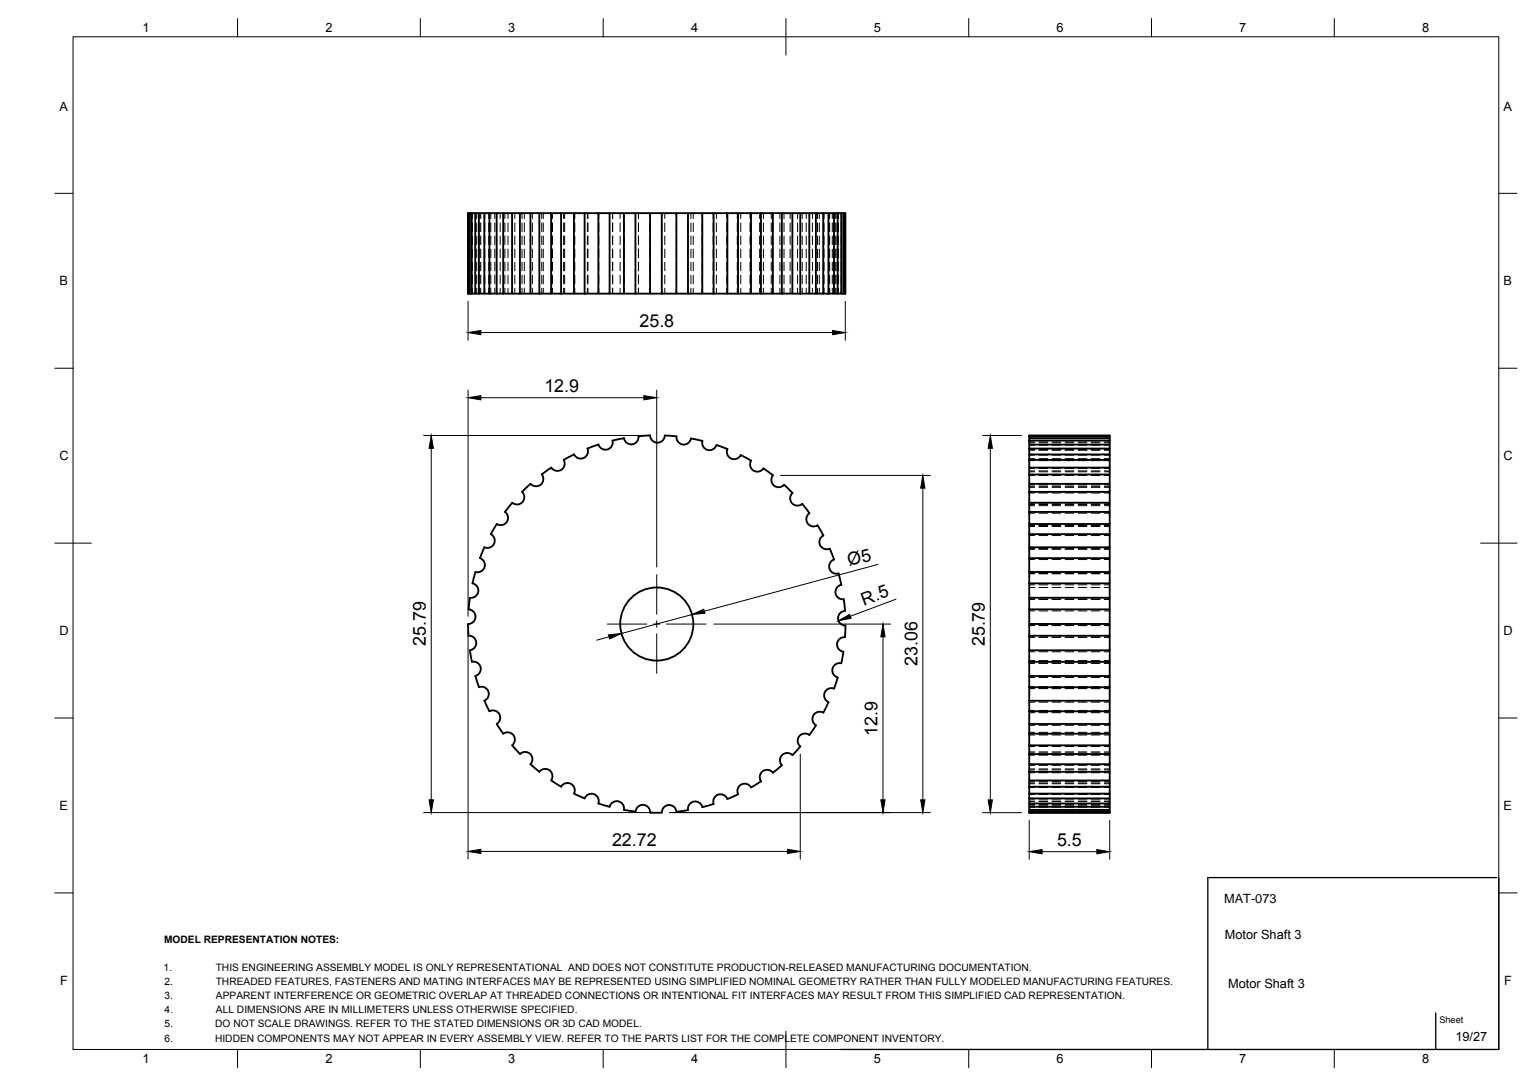
ISO-10303-21;
HEADER;
/* Generated by software containing ST-Developer
 * from STEP Tools, Inc. (www.steptools.com) 
 */

FILE_DESCRIPTION(
/* description */ ('CAx-IF Rec.Pracs.---Representation and Presentation of Product Manufa
cturing Information (PMI)---4.0---2014-10-13'),
/* implementation_level */ '2;1');

FILE_NAME(
/* name */ 'Motor Shaft 3.step',
/* time_stamp */ '2026-10-24T18:52:33-07:00',
/* author */ (''),
/* organization */ (''),
/* preprocessor_version */ 'ST-DEVELOPER v20.2',
/* originating_system */ 'Autodesk Translation Framework v15.17.0.0',
/* authorisation */ '');

FILE_SCHEMA (('AP242_MANAGED_MODEL_BASED_3D_ENGINEERING_MIM_LF { 1 0 10303 442 2 1 4 }'));
ENDSEC;

DATA;
#10=MECHANICAL_DESIGN_GEOMETRIC_PRESENTATION_REPRESENTATION('',(#434),#34876);
#368=SHAPE_REPRESENTATION_RELATIONSHIP('SRR','None',#35005,#401);
#401=ADVANCED_BREP_SHAPE_REPRESENTATION('',(#467),#34863);
#434=STYLED_ITEM('',(#35161),#467);
#467=MANIFOLD_SOLID_BREP('Motor Shaft 3',#19574);
#558=FACE_BOUND('',#6621,.T.);
#559=FACE_BOUND('',#6668,.T.);
#925=PLANE('',#21507);
#926=PLANE('',#21645);
#2083=LINE('',#32384,#3682);
#2084=LINE('',#32388,#3683);
#2085=LINE('',#32393,#3684);
#2086=LINE('',#32397,#3685);
#2087=LINE('',#32402,#3686);
#2088=LINE('',#32406,#3687);
#2089=LINE('',#32411,#3688);
#2090=LINE('',#32415,#3689);
#2091=LINE('',#32420,#3690);
#2092=LINE('',#32424,#3691);
#2093=LINE('',#32429,#3692);
#2094=LINE('',#32433,#3693);
#2095=LINE('',#32438,#3694);
#2096=LINE('',#32442,#3695);
#2097=LINE('',#32447,#3696);
#2098=LINE('',#32451,#3697);
#2099=LINE('',#32456,#3698);
#2100=LINE('',#32460,#3699);
#2101=LINE('',#32465,#3700);
#2102=LINE('',#32469,#3701);
#2103=LINE('',#32474,#3702);
#2104=LINE('',#32478,#3703);
#2105=LINE('',#32483,#3704);
#2106=LINE('',#32487,#3705);
#2107=LINE('',#32492,#3706);
#2108=LINE('',#32496,#3707);
#2109=LINE('',#32501,#3708);
#2110=LINE('',#32505,#3709);
#2111=LINE('',#32510,#3710);
#2112=LINE('',#32514,#3711);
#2113=LINE('',#32519,#3712);
#2114=LINE('',#32523,#3713);
#2115=LINE('',#32528,#3714);
#2116=LINE('',#32532,#3715);
#2117=LINE('',#32537,#3716);
#2118=LINE('',#32541,#3717);
#2119=LINE('',#32546,#3718);
#2120=LINE('',#32550,#3719);
#2121=LINE('',#32555,#3720);
#2122=LINE('',#32559,#3721);
#2123=LINE('',#32564,#3722);
#2124=LINE('',#32568,#3723);
#2125=LINE('',#32573,#3724);
#2126=LINE('',#32577,#3725);
#2127=LINE('',#32582,#3726);
#2128=LINE('',#32586,#3727);
#2129=LINE('',#32591,#3728);
#2130=LINE('',#32595,#3729);
#2131=LINE('',#32600,#3730);
#2132=LINE('',#32604,#3731);
#2133=LINE('',#32609,#3732);
#2134=LINE('',#32613,#3733);
#2135=LINE('',#32618,#3734);
#2136=LINE('',#32622,#3735);
#2137=LINE('',#32627,#3736);
#2138=LINE('',#32631,#3737);
#2139=LINE('',#32636,#3738);
#2140=LINE('',#32640,#3739);
#2141=LINE('',#32645,#3740);
#2142=LINE('',#32649,#3741);
#2143=LINE('',#32654,#3742);
#2144=LINE('',#32658,#3743);
#2145=LINE('',#32663,#3744);
#2146=LINE('',#32667,#3745);
#2147=LINE('',#32672,#3746);
#2148=LINE('',#32676,#3747);
#2149=LINE('',#32681,#3748);
#2150=LINE('',#32685,#3749);
#2151=LINE('',#32690,#3750);
#2152=LINE('',#32694,#3751);
#2153=LINE('',#32699,#3752);
#2154=LINE('',#32703,#3753);
#2155=LINE('',#32708,#3754);
#2156=LINE('',#32712,#3755);
#2157=LINE('',#32717,#3756);
#2158=LINE('',#32721,#3757);
#2159=LINE('',#32726,#3758);
#2160=LINE('',#32730,#3759);
#2161=LINE('',#32735,#3760);
#2162=LINE('',#32739,#3761);
#2163=LINE('',#32744,#3762);
#2164=LINE('',#32748,#3763);
#2165=LINE('',#32753,#3764);
#2166=LINE('',#32757,#3765);
#2167=LINE('',#32762,#3766);
#2168=LINE('',#32766,#3767);
#2169=LINE('',#32771,#3768);
#2170=LINE('',#32775,#3769);
#2171=LINE('',#32831,#3770);
#2172=LINE('',#32834,#3771);
#2173=LINE('',#32928,#3772);
#3682=VECTOR('',#26108,1.);
#3683=VECTOR('',#26111,1.);
#3684=VECTOR('',#26116,1.);
#3685=VECTOR('',#26119,1.);
#3686=VECTOR('',#26124,1.);
#3687=VECTOR('',#26127,1.);
#3688=VECTOR('',#26132,1.);
#3689=VECTOR('',#26135,1.);
#3690=VECTOR('',#26140,1.);
#3691=VECTOR('',#26143,1.);
#3692=VECTOR('',#26148,1.);
#3693=VECTOR('',#26151,1.);
#3694=VECTOR('',#26156,1.);
#3695=VECTOR('',#26159,1.);
#3696=VECTOR('',#26164,1.);
#3697=VECTOR('',#26167,1.);
#3698=VECTOR('',#26172,1.);
#3699=VECTOR('',#26175,1.);
#3700=VECTOR('',#26180,1.);
#3701=VECTOR('',#26183,1.);
#3702=VECTOR('',#26188,1.);
#3703=VECTOR('',#26191,1.);
#3704=VECTOR('',#26196,1.);
#3705=VECTOR('',#26199,1.);
#3706=VECTOR('',#26204,1.);
#3707=VECTOR('',#26207,1.);
#3708=VECTOR('',#26212,1.);
#3709=VECTOR('',#26215,1.);
#3710=VECTOR('',#26220,1.);
#3711=VECTOR('',#26223,1.);
#3712=VECTOR('',#26228,1.);
#3713=VECTOR('',#26231,1.);
#3714=VECTOR('',#26236,1.);
#3715=VECTOR('',#26239,1.);
#3716=VECTOR('',#26244,1.);
#3717=VECTOR('',#26247,1.);
#3718=VECTOR('',#26252,1.);
#3719=VECTOR('',#26255,1.);
#3720=VECTOR('',#26260,1.);
#3721=VECTOR('',#26263,1.);
#3722=VECTOR('',#26268,1.);
#3723=VECTOR('',#26271,1.);
#3724=VECTOR('',#26276,1.);
#3725=VECTOR('',#26279,1.);
#3726=VECTOR('',#26284,1.);
#3727=VECTOR('',#26287,1.);
#3728=VECTOR('',#26292,1.);
#3729=VECTOR('',#26295,1.);
#3730=VECTOR('',#26300,1.);
#3731=VECTOR('',#26303,1.);
#3732=VECTOR('',#26308,1.);
#3733=VECTOR('',#26311,1.);
#3734=VECTOR('',#26316,1.);
#3735=VECTOR('',#26319,1.);
#3736=VECTOR('',#26324,1.);
#3737=VECTOR('',#26327,1.);
#3738=VECTOR('',#26332,1.);
#3739=VECTOR('',#26335,1.);
#3740=VECTOR('',#26340,1.);
#3741=VECTOR('',#26343,1.);
#3742=VECTOR('',#26348,1.);
#3743=VECTOR('',#26351,1.);
#3744=VECTOR('',#26356,1.);
#3745=VECTOR('',#26359,1.);
#3746=VECTOR('',#26364,1.);
#3747=VECTOR('',#26367,1.);
#3748=VECTOR('',#26372,1.);
#3749=VECTOR('',#26375,1.);
#3750=VECTOR('',#26380,1.);
#3751=VECTOR('',#26383,1.);
#3752=VECTOR('',#26388,1.);
#3753=VECTOR('',#26391,1.);
#3754=VECTOR('',#26396,1.);
#3755=VECTOR('',#26399,1.);
#3756=VECTOR('',#26404,1.);
#3757=VECTOR('',#26407,1.);
#3758=VECTOR('',#26412,1.);
#3759=VECTOR('',#26415,1.);
#3760=VECTOR('',#26420,1.);
#3761=VECTOR('',#26423,1.);
#3762=VECTOR('',#26428,1.);
#3763=VECTOR('',#26431,1.);
#3764=VECTOR('',#26436,1.);
#3765=VECTOR('',#26439,1.);
#3766=VECTOR('',#26444,1.);
#3767=VECTOR('',#26447,1.);
#3768=VECTOR('',#26452,1.);
#3769=VECTOR('',#26455,1.);
#3770=VECTOR('',#26558,1.);
#3771=VECTOR('',#26561,1.);
#3772=VECTOR('',#26746,0.0025);
#4588=CYLINDRICAL_SURFACE('',#21375,0.0005);
#4589=CYLINDRICAL_SURFACE('',#21378,0.0005);
#4590=CYLINDRICAL_SURFACE('',#21381,0.0005);
#4591=CYLINDRICAL_SURFACE('',#21384,0.0005);
#4592=CYLINDRICAL_SURFACE('',#21387,0.0005);
#4593=CYLINDRICAL_SURFACE('',#21390,0.0005);
#4594=CYLINDRICAL_SURFACE('',#21393,0.0005);
#4595=CYLINDRICAL_SURFACE('',#21396,0.0005);
#4596=CYLINDRICAL_SURFACE('',#21399,0.0005);
#4597=CYLINDRICAL_SURFACE('',#21402,0.0005);
#4598=CYLINDRICAL_SURFACE('',#21405,0.0005);
#4599=CYLINDRICAL_SURFACE('',#21408,0.0005);
#4600=CYLINDRICAL_SURFACE('',#21411,0.0005);
#4601=CYLINDRICAL_SURFACE('',#21414,0.0005);
#4602=CYLINDRICAL_SURFACE('',#21417,0.0005);
#4603=CYLINDRICAL_SURFACE('',#21420,0.0005);
#4604=CYLINDRICAL_SURFACE('',#21423,0.0005);
#4605=CYLINDRICAL_SURFACE('',#21426,0.0005);
#4606=CYLINDRICAL_SURFACE('',#21429,0.0005);
#4607=CYLINDRICAL_SURFACE('',#21432,0.0005);
#4608=CYLINDRICAL_SURFACE('',#21435,0.0005);
#4609=CYLINDRICAL_SURFACE('',#21438,0.0005);
#4610=CYLINDRICAL_SURFACE('',#21441,0.0005);
#4611=CYLINDRICAL_SURFACE('',#21444,0.0005);
#4612=CYLINDRICAL_SURFACE('',#21447,0.0005);
#4613=CYLINDRICAL_SURFACE('',#21450,0.0005);
#4614=CYLINDRICAL_SURFACE('',#21453,0.0005);
#4615=CYLINDRICAL_SURFACE('',#21456,0.0005);
#4616=CYLINDRICAL_SURFACE('',#21459,0.0005);
#4617=CYLINDRICAL_SURFACE('',#21462,0.0005);
#4618=CYLINDRICAL_SURFACE('',#21465,0.0005);
#4619=CYLINDRICAL_SURFACE('',#21468,0.0005);
#4620=CYLINDRICAL_SURFACE('',#21471,0.0005);
#4621=CYLINDRICAL_SURFACE('',#21474,0.0005);
#4622=CYLINDRICAL_SURFACE('',#21477,0.0005);
#4623=CYLINDRICAL_SURFACE('',#21480,0.0005);
#4624=CYLINDRICAL_SURFACE('',#21483,0.0005);
#4625=CYLINDRICAL_SURFACE('',#21486,0.0005);
#4626=CYLINDRICAL_SURFACE('',#21489,0.0005);
#4627=CYLINDRICAL_SURFACE('',#21492,0.0005);
#4628=CYLINDRICAL_SURFACE('',#21495,0.0005);
#4629=CYLINDRICAL_SURFACE('',#21498,0.0005);
#4630=CYLINDRICAL_SURFACE('',#21501,0.0005);
#4631=CYLINDRICAL_SURFACE('',#21504,0.0005);
#4632=CYLINDRICAL_SURFACE('',#21555,0.0129);
#4633=CYLINDRICAL_SURFACE('',#21557,0.0129);
#4634=CYLINDRICAL_SURFACE('',#21559,0.0129);
#4635=CYLINDRICAL_SURFACE('',#21561,0.0129);
#4636=CYLINDRICAL_SURFACE('',#21563,0.0129);
#4637=CYLINDRICAL_SURFACE('',#21565,0.0129);
#4638=CYLINDRICAL_SURFACE('',#21567,0.0129);
#4639=CYLINDRICAL_SURFACE('',#21569,0.0129);
#4640=CYLINDRICAL_SURFACE('',#21571,0.0129);
#4641=CYLINDRICAL_SURFACE('',#21573,0.0129);
#4642=CYLINDRICAL_SURFACE('',#21575,0.0129);
#4643=CYLINDRICAL_SURFACE('',#21577,0.0129);
#4644=CYLINDRICAL_SURFACE('',#21579,0.0129);
#4645=CYLINDRICAL_SURFACE('',#21581,0.0129);
#4646=CYLINDRICAL_SURFACE('',#21583,0.0129);
#4647=CYLINDRICAL_SURFACE('',#21585,0.0129);
#4648=CYLINDRICAL_SURFACE('',#21587,0.0129);
#4649=CYLINDRICAL_SURFACE('',#21589,0.0129);
#4650=CYLINDRICAL_SURFACE('',#21591,0.0129);
#4651=CYLINDRICAL_SURFACE('',#21593,0.0129);
#4652=CYLINDRICAL_SURFACE('',#21595,0.0129);
#4653=CYLINDRICAL_SURFACE('',#21597,0.0129);
#4654=CYLINDRICAL_SURFACE('',#21599,0.0129);
#4655=CYLINDRICAL_SURFACE('',#21601,0.0129);
#4656=CYLINDRICAL_SURFACE('',#21603,0.0129);
#4657=CYLINDRICAL_SURFACE('',#21605,0.0129);
#4658=CYLINDRICAL_SURFACE('',#21607,0.0129);
#4659=CYLINDRICAL_SURFACE('',#21609,0.0129);
#4660=CYLINDRICAL_SURFACE('',#21611,0.0129);
#4661=CYLINDRICAL_SURFACE('',#21613,0.0129);
#4662=CYLINDRICAL_SURFACE('',#21615,0.0129);
#4663=CYLINDRICAL_SURFACE('',#21617,0.0129);
#4664=CYLINDRICAL_SURFACE('',#21619,0.0129);
#4665=CYLINDRICAL_SURFACE('',#21621,0.0129);
#4666=CYLINDRICAL_SURFACE('',#21623,0.0129);
#4667=CYLINDRICAL_SURFACE('',#21625,0.0129);
#4668=CYLINDRICAL_SURFACE('',#21627,0.0129);
#4669=CYLINDRICAL_SURFACE('',#21629,0.0129);
#4670=CYLINDRICAL_SURFACE('',#21631,0.0129);
#4671=CYLINDRICAL_SURFACE('',#21633,0.0129);
#4672=CYLINDRICAL_SURFACE('',#21635,0.0129);
#4673=CYLINDRICAL_SURFACE('',#21637,0.0129);
#4674=CYLINDRICAL_SURFACE('',#21639,0.0129);
#4675=CYLINDRICAL_SURFACE('',#21641,0.0129);
#4676=CYLINDRICAL_SURFACE('',#21643,0.0005);
#4677=CYLINDRICAL_SURFACE('',#21648,0.0129);
#4678=CYLINDRICAL_SURFACE('',#21649,0.0025);
#5453=FACE_OUTER_BOUND('',#6576,.T.);
#5454=FACE_OUTER_BOUND('',#6577,.T.);
#5455=FACE_OUTER_BOUND('',#6578,.T.);
#5456=FACE_OUTER_BOUND('',#6579,.T.);
#5457=FACE_OUTER_BOUND('',#6580,.T.);
#5458=FACE_OUTER_BOUND('',#6581,.T.);
#5459=FACE_OUTER_BOUND('',#6582,.T.);
#5460=FACE_OUTER_BOUND('',#6583,.T.);
#5461=FACE_OUTER_BOUND('',#6584,.T.);
#5462=FACE_OUTER_BOUND('',#6585,.T.);
#5463=FACE_OUTER_BOUND('',#6586,.T.);
#5464=FACE_OUTER_BOUND('',#6587,.T.);
#5465=FACE_OUTER_BOUND('',#6588,.T.);
#5466=FACE_OUTER_BOUND('',#6589,.T.);
#5467=FACE_OUTER_BOUND('',#6590,.T.);
#5468=FACE_OUTER_BOUND('',#6591,.T.);
#5469=FACE_OUTER_BOUND('',#6592,.T.);
#5470=FACE_OUTER_BOUND('',#6593,.T.);
#5471=FACE_OUTER_BOUND('',#6594,.T.);
#5472=FACE_OUTER_BOUND('',#6595,.T.);
#5473=FACE_OUTER_BOUND('',#6596,.T.);
#5474=FACE_OUTER_BOUND('',#6597,.T.);
#5475=FACE_OUTER_BOUND('',#6598,.T.);
#5476=FACE_OUTER_BOUND('',#6599,.T.);
#5477=FACE_OUTER_BOUND('',#6600,.T.);
#5478=FACE_OUTER_BOUND('',#6601,.T.);
#5479=FACE_OUTER_BOUND('',#6602,.T.);
#5480=FACE_OUTER_BOUND('',#6603,.T.);
#5481=FACE_OUTER_BOUND('',#6604,.T.);
#5482=FACE_OUTER_BOUND('',#6605,.T.);
#5483=FACE_OUTER_BOUND('',#6606,.T.);
#5484=FACE_OUTER_BOUND('',#6607,.T.);
#5485=FACE_OUTER_BOUND('',#6608,.T.);
#5486=FACE_OUTER_BOUND('',#6609,.T.);
#5487=FACE_OUTER_BOUND('',#6610,.T.);
#5488=FACE_OUTER_BOUND('',#6611,.T.);
#5489=FACE_OUTER_BOUND('',#6612,.T.);
#5490=FACE_OUTER_BOUND('',#6613,.T.);
#5491=FACE_OUTER_BOUND('',#6614,.T.);
#5492=FACE_OUTER_BOUND('',#6615,.T.);
#5493=FACE_OUTER_BOUND('',#6616,.T.);
#5494=FACE_OUTER_BOUND('',#6617,.T.);
#5495=FACE_OUTER_BOUND('',#6618,.T.);
#5496=FACE_OUTER_BOUND('',#6619,.T.);
#5497=FACE_OUTER_BOUND('',#6620,.T.);
#5498=FACE_OUTER_BOUND('',#6622,.T.);
#5499=FACE_OUTER_BOUND('',#6623,.T.);
#5500=FACE_OUTER_BOUND('',#6624,.T.);
#5501=FACE_OUTER_BOUND('',#6625,.T.);
#5502=FACE_OUTER_BOUND('',#6626,.T.);
#5503=FACE_OUTER_BOUND('',#6627,.T.);
#5504=FACE_OUTER_BOUND('',#6628,.T.);
#5505=FACE_OUTER_BOUND('',#6629,.T.);
#5506=FACE_OUTER_BOUND('',#6630,.T.);
#5507=FACE_OUTER_BOUND('',#6631,.T.);
#5508=FACE_OUTER_BOUND('',#6632,.T.);
#5509=FACE_OUTER_BOUND('',#6633,.T.);
#5510=FACE_OUTER_BOUND('',#6634,.T.);
#5511=FACE_OUTER_BOUND('',#6635,.T.);
#5512=FACE_OUTER_BOUND('',#6636,.T.);
#5513=FACE_OUTER_BOUND('',#6637,.T.);
#5514=FACE_OUTER_BOUND('',#6638,.T.);
#5515=FACE_OUTER_BOUND('',#6639,.T.);
#5516=FACE_OUTER_BOUND('',#6640,.T.);
#5517=FACE_OUTER_BOUND('',#6641,.T.);
#5518=FACE_OUTER_BOUND('',#6642,.T.);
#5519=FACE_OUTER_BOUND('',#6643,.T.);
#5520=FACE_OUTER_BOUND('',#6644,.T.);
#5521=FACE_OUTER_BOUND('',#6645,.T.);
#5522=FACE_OUTER_BOUND('',#6646,.T.);
#5523=FACE_OUTER_BOUND('',#6647,.T.);
#5524=FACE_OUTER_BOUND('',#6648,.T.);
#5525=FACE_OUTER_BOUND('',#6649,.T.);
#5526=FACE_OUTER_BOUND('',#6650,.T.);
#5527=FACE_OUTER_BOUND('',#6651,.T.);
#5528=FACE_OUTER_BOUND('',#6652,.T.);
#5529=FACE_OUTER_BOUND('',#6653,.T.);
#5530=FACE_OUTER_BOUND('',#6654,.T.);
#5531=FACE_OUTER_BOUND('',#6655,.T.);
#5532=FACE_OUTER_BOUND('',#6656,.T.);
#5533=FACE_OUTER_BOUND('',#6657,.T.);
#5534=FACE_OUTER_BOUND('',#6658,.T.);
#5535=FACE_OUTER_BOUND('',#6659,.T.);
#5536=FACE_OUTER_BOUND('',#6660,.T.);
#5537=FACE_OUTER_BOUND('',#6661,.T.);
#5538=FACE_OUTER_BOUND('',#6662,.T.);
#5539=FACE_OUTER_BOUND('',#6663,.T.);
#5540=FACE_OUTER_BOUND('',#6664,.T.);
#5541=FACE_OUTER_BOUND('',#6665,.T.);
#5542=FACE_OUTER_BOUND('',#6666,.T.);
#5543=FACE_OUTER_BOUND('',#6667,.T.);
#5544=FACE_OUTER_BOUND('',#6669,.T.);
#5545=FACE_OUTER_BOUND('',#6670,.T.);
#6576=EDGE_LOOP('',(#16334,#16335,#16336,#16337));
#6577=EDGE_LOOP('',(#16338,#16339,#16340,#16341));
#6578=EDGE_LOOP('',(#16342,#16343,#16344,#16345));
#6579=EDGE_LOOP('',(#16346,#16347,#16348,#16349));
#6580=EDGE_LOOP('',(#16350,#16351,#16352,#16353));
#6581=EDGE_LOOP('',(#16354,#16355,#16356,#16357));
#6582=EDGE_LOOP('',(#16358,#16359,#16360,#16361));
#6583=EDGE_LOOP('',(#16362,#16363,#16364,#16365));
#6584=EDGE_LOOP('',(#16366,#16367,#16368,#16369));
#6585=EDGE_LOOP('',(#16370,#16371,#16372,#16373));
#6586=EDGE_LOOP('',(#16374,#16375,#16376,#16377));
#6587=EDGE_LOOP('',(#16378,#16379,#16380,#16381));
#6588=EDGE_LOOP('',(#16382,#16383,#16384,#16385));
#6589=EDGE_LOOP('',(#16386,#16387,#16388,#16389));
#6590=EDGE_LOOP('',(#16390,#16391,#16392,#16393));
#6591=EDGE_LOOP('',(#16394,#16395,#16396,#16397));
#6592=EDGE_LOOP('',(#16398,#16399,#16400,#16401));
#6593=EDGE_LOOP('',(#16402,#16403,#16404,#16405));
#6594=EDGE_LOOP('',(#16406,#16407,#16408,#16409));
#6595=EDGE_LOOP('',(#16410,#16411,#16412,#16413));
#6596=EDGE_LOOP('',(#16414,#16415,#16416,#16417));
#6597=EDGE_LOOP('',(#16418,#16419,#16420,#16421));
#6598=EDGE_LOOP('',(#16422,#16423,#16424,#16425));
#6599=EDGE_LOOP('',(#16426,#16427,#16428,#16429));
#6600=EDGE_LOOP('',(#16430,#16431,#16432,#16433));
#6601=EDGE_LOOP('',(#16434,#16435,#16436,#16437));
#6602=EDGE_LOOP('',(#16438,#16439,#16440,#16441));
#6603=EDGE_LOOP('',(#16442,#16443,#16444,#16445));
#6604=EDGE_LOOP('',(#16446,#16447,#16448,#16449));
#6605=EDGE_LOOP('',(#16450,#16451,#16452,#16453));
#6606=EDGE_LOOP('',(#16454,#16455,#16456,#16457));
#6607=EDGE_LOOP('',(#16458,#16459,#16460,#16461));
#6608=EDGE_LOOP('',(#16462,#16463,#16464,#16465));
#6609=EDGE_LOOP('',(#16466,#16467,#16468,#16469));
#6610=EDGE_LOOP('',(#16470,#16471,#16472,#16473));
#6611=EDGE_LOOP('',(#16474,#16475,#16476,#16477));
#6612=EDGE_LOOP('',(#16478,#16479,#16480,#16481));
#6613=EDGE_LOOP('',(#16482,#16483,#16484,#16485));
#6614=EDGE_LOOP('',(#16486,#16487,#16488,#16489));
#6615=EDGE_LOOP('',(#16490,#16491,#16492,#16493));
#6616=EDGE_LOOP('',(#16494,#16495,#16496,#16497));
#6617=EDGE_LOOP('',(#16498,#16499,#16500,#16501));
#6618=EDGE_LOOP('',(#16502,#16503,#16504,#16505));
#6619=EDGE_LOOP('',(#16506,#16507,#16508,#16509));
#6620=EDGE_LOOP('',(#16510,#16511,#16512,#16513,#16514,#16515,#16516,#16517,
#16518,#16519,#16520,#16521,#16522,#16523,#16524,#16525,#16526,#16527,#16528,
#16529,#16530,#16531,#16532,#16533,#16534,#16535,#16536,#16537,#16538,#16539,
#16540,#16541,#16542,#16543,#16544,#16545,#16546,#16547,#16548,#16549,#16550,
#16551,#16552,#16553,#16554,#16555,#16556,#16557,#16558,#16559,#16560,#16561,
#16562,#16563,#16564,#16565,#16566,#16567,#16568,#16569,#16570,#16571,#16572,
#16573,#16574,#16575,#16576,#16577,#16578,#16579,#16580,#16581,#16582,#16583,
#16584,#16585,#16586,#16587,#16588,#16589,#16590,#16591,#16592,#16593,#16594,
#16595,#16596,#16597,#16598,#16599));
#6621=EDGE_LOOP('',(#16600));
#6622=EDGE_LOOP('',(#16601,#16602,#16603,#16604));
#6623=EDGE_LOOP('',(#16605,#16606,#16607,#16608));
#6624=EDGE_LOOP('',(#16609,#16610,#16611,#16612));
#6625=EDGE_LOOP('',(#16613,#16614,#16615,#16616));
#6626=EDGE_LOOP('',(#16617,#16618,#16619,#16620));
#6627=EDGE_LOOP('',(#16621,#16622,#16623,#16624));
#6628=EDGE_LOOP('',(#16625,#16626,#16627,#16628));
#6629=EDGE_LOOP('',(#16629,#16630,#16631,#16632));
#6630=EDGE_LOOP('',(#16633,#16634,#16635,#16636));
#6631=EDGE_LOOP('',(#16637,#16638,#16639,#16640));
#6632=EDGE_LOOP('',(#16641,#16642,#16643,#16644));
#6633=EDGE_LOOP('',(#16645,#16646,#16647,#16648));
#6634=EDGE_LOOP('',(#16649,#16650,#16651,#16652));
#6635=EDGE_LOOP('',(#16653,#16654,#16655,#16656));
#6636=EDGE_LOOP('',(#16657,#16658,#16659,#16660));
#6637=EDGE_LOOP('',(#16661,#16662,#16663,#16664));
#6638=EDGE_LOOP('',(#16665,#16666,#16667,#16668));
#6639=EDGE_LOOP('',(#16669,#16670,#16671,#16672));
#6640=EDGE_LOOP('',(#16673,#16674,#16675,#16676));
#6641=EDGE_LOOP('',(#16677,#16678,#16679,#16680));
#6642=EDGE_LOOP('',(#16681,#16682,#16683,#16684));
#6643=EDGE_LOOP('',(#16685,#16686,#16687,#16688));
#6644=EDGE_LOOP('',(#16689,#16690,#16691,#16692));
#6645=EDGE_LOOP('',(#16693,#16694,#16695,#16696));
#6646=EDGE_LOOP('',(#16697,#16698,#16699,#16700));
#6647=EDGE_LOOP('',(#16701,#16702,#16703,#16704));
#6648=EDGE_LOOP('',(#16705,#16706,#16707,#16708));
#6649=EDGE_LOOP('',(#16709,#16710,#16711,#16712));
#6650=EDGE_LOOP('',(#16713,#16714,#16715,#16716));
#6651=EDGE_LOOP('',(#16717,#16718,#16719,#16720));
#6652=EDGE_LOOP('',(#16721,#16722,#16723,#16724));
#6653=EDGE_LOOP('',(#16725,#16726,#16727,#16728));
#6654=EDGE_LOOP('',(#16729,#16730,#16731,#16732));
#6655=EDGE_LOOP('',(#16733,#16734,#16735,#16736));
#6656=EDGE_LOOP('',(#16737,#16738,#16739,#16740));
#6657=EDGE_LOOP('',(#16741,#16742,#16743,#16744));
#6658=EDGE_LOOP('',(#16745,#16746,#16747,#16748));
#6659=EDGE_LOOP('',(#16749,#16750,#16751,#16752));
#6660=EDGE_LOOP('',(#16753,#16754,#16755,#16756));
#6661=EDGE_LOOP('',(#16757,#16758,#16759,#16760));
#6662=EDGE_LOOP('',(#16761,#16762,#16763,#16764));
#6663=EDGE_LOOP('',(#16765,#16766,#16767,#16768));
#6664=EDGE_LOOP('',(#16769,#16770,#16771,#16772));
#6665=EDGE_LOOP('',(#16773,#16774,#16775,#16776));
#6666=EDGE_LOOP('',(#16777,#16778,#16779,#16780));
#6667=EDGE_LOOP('',(#16781,#16782,#16783,#16784,#16785,#16786,#16787,#16788,
#16789,#16790,#16791,#16792,#16793,#16794,#16795,#16796,#16797,#16798,#16799,
#16800,#16801,#16802,#16803,#16804,#16805,#16806,#16807,#16808,#16809,#16810,
#16811,#16812,#16813,#16814,#16815,#16816,#16817,#16818,#16819,#16820,#16821,
#16822,#16823,#16824,#16825,#16826,#16827,#16828,#16829,#16830,#16831,#16832,
#16833,#16834,#16835,#16836,#16837,#16838,#16839,#16840,#16841,#16842,#16843,
#16844,#16845,#16846,#16847,#16848,#16849,#16850,#16851,#16852,#16853,#16854,
#16855,#16856,#16857,#16858,#16859,#16860,#16861,#16862,#16863,#16864,#16865,
#16866,#16867,#16868,#16869,#16870));
#6668=EDGE_LOOP('',(#16871));
#6669=EDGE_LOOP('',(#16872,#16873,#16874,#16875));
#6670=EDGE_LOOP('',(#16876,#16877,#16878,#16879));
#7623=CIRCLE('',#21376,0.000500000000011295);
#7624=CIRCLE('',#21377,0.000500000000011295);
#7625=CIRCLE('',#21379,0.000500000000012369);
#7626=CIRCLE('',#21380,0.000500000000012369);
#7627=CIRCLE('',#21382,0.000500000000013203);
#7628=CIRCLE('',#21383,0.000500000000013203);
#7629=CIRCLE('',#21385,0.00050000000001378);
#7630=CIRCLE('',#21386,0.00050000000001378);
#7631=CIRCLE('',#21388,0.000500000000014088);
#7632=CIRCLE('',#21389,0.000500000000014088);
#7633=CIRCLE('',#21391,0.000500000000014123);
#7634=CIRCLE('',#21392,0.000500000000014123);
#7635=CIRCLE('',#21394,0.000500000000013882);
#7636=CIRCLE('',#21395,0.000500000000013882);
#7637=CIRCLE('',#21397,0.000500000000013372);
#7638=CIRCLE('',#21398,0.000500000000013372);
#7639=CIRCLE('',#21400,0.000500000000012601);
#7640=CIRCLE('',#21401,0.000500000000012601);
#7641=CIRCLE('',#21403,0.000500000000011585);
#7642=CIRCLE('',#21404,0.000500000000011585);
#7643=CIRCLE('',#21406,0.000500000000010343);
#7644=CIRCLE('',#21407,0.000500000000010343);
#7645=CIRCLE('',#21409,0.000500000000010991);
#7646=CIRCLE('',#21410,0.000500000000010991);
#7647=CIRCLE('',#21412,0.000500000000012122);
#7648=CIRCLE('',#21413,0.000500000000012122);
#7649=CIRCLE('',#21415,0.000500000000013018);
#7650=CIRCLE('',#21416,0.000500000000013018);
#7651=CIRCLE('',#21418,0.00050000000001366);
#7652=CIRCLE('',#21419,0.00050000000001366);
#7653=CIRCLE('',#21421,0.000500000000014037);
#7654=CIRCLE('',#21422,0.000500000000014037);
#7655=CIRCLE('',#21424,0.00050000000001414);
#7656=CIRCLE('',#21425,0.00050000000001414);
#7657=CIRCLE('',#21427,0.000500000000013968);
#7658=CIRCLE('',#21428,0.000500000000013968);
#7659=CIRCLE('',#21430,0.000500000000013524);
#7660=CIRCLE('',#21431,0.000500000000013524);
#7661=CIRCLE('',#21433,0.000500000000012817);
#7662=CIRCLE('',#21434,0.000500000000012817);
#7663=CIRCLE('',#21436,0.000500000000011861);
#7664=CIRCLE('',#21437,0.000500000000011861);
#7665=CIRCLE('',#21439,0.000500000000010673);
#7666=CIRCLE('',#21440,0.000500000000010673);
#7667=CIRCLE('',#21442,0.000500000000010673);
#7668=CIRCLE('',#21443,0.000500000000010673);
#7669=CIRCLE('',#21445,0.000500000000011861);
#7670=CIRCLE('',#21446,0.000500000000011861);
#7671=CIRCLE('',#21448,0.000500000000012817);
#7672=CIRCLE('',#21449,0.000500000000012817);
#7673=CIRCLE('',#21451,0.000500000000013524);
#7674=CIRCLE('',#21452,0.000500000000013524);
#7675=CIRCLE('',#21454,0.000500000000013968);
#7676=CIRCLE('',#21455,0.000500000000013968);
#7677=CIRCLE('',#21457,0.00050000000001414);
#7678=CIRCLE('',#21458,0.00050000000001414);
#7679=CIRCLE('',#21460,0.000500000000014037);
#7680=CIRCLE('',#21461,0.000500000000014037);
#7681=CIRCLE('',#21463,0.00050000000001366);
#7682=CIRCLE('',#21464,0.00050000000001366);
#7683=CIRCLE('',#21466,0.000500000000013018);
#7684=CIRCLE('',#21467,0.000500000000013018);
#7685=CIRCLE('',#21469,0.000500000000012122);
#7686=CIRCLE('',#21470,0.000500000000012122);
#7687=CIRCLE('',#21472,0.000500000000010991);
#7688=CIRCLE('',#21473,0.000500000000010991);
#7689=CIRCLE('',#21475,0.000500000000010343);
#7690=CIRCLE('',#21476,0.000500000000010343);
#7691=CIRCLE('',#21478,0.000500000000011585);
#7692=CIRCLE('',#21479,0.000500000000011585);
#7693=CIRCLE('',#21481,0.000500000000012601);
#7694=CIRCLE('',#21482,0.000500000000012601);
#7695=CIRCLE('',#21484,0.000500000000013372);
#7696=CIRCLE('',#21485,0.000500000000013372);
#7697=CIRCLE('',#21487,0.000500000000013882);
#7698=CIRCLE('',#21488,0.000500000000013882);
#7699=CIRCLE('',#21490,0.000500000000014123);
#7700=CIRCLE('',#21491,0.000500000000014123);
#7701=CIRCLE('',#21493,0.000500000000014088);
#7702=CIRCLE('',#21494,0.000500000000014088);
#7703=CIRCLE('',#21496,0.00050000000001378);
#7704=CIRCLE('',#21497,0.00050000000001378);
#7705=CIRCLE('',#21499,0.000500000000013203);
#7706=CIRCLE('',#21500,0.000500000000013203);
#7707=CIRCLE('',#21502,0.000500000000012369);
#7708=CIRCLE('',#21503,0.000500000000012369);
#7709=CIRCLE('',#21505,0.000500000000011295);
#7710=CIRCLE('',#21506,0.000500000000011295);
#7711=CIRCLE('',#21508,0.01290000000001);
#7712=CIRCLE('',#21509,0.00050000000001);
#7713=CIRCLE('',#21510,0.01290000000001);
#7714=CIRCLE('',#21511,0.01290000000001);
#7715=CIRCLE('',#21512,0.01290000000001);
#7716=CIRCLE('',#21513,0.01290000000001);
#7717=CIRCLE('',#21514,0.01290000000001);
#7718=CIRCLE('',#21515,0.01290000000001);
#7719=CIRCLE('',#21516,0.01290000000001);
#7720=CIRCLE('',#21517,0.01290000000001);
#7721=CIRCLE('',#21518,0.01290000000001);
#7722=CIRCLE('',#21519,0.01290000000001);
#7723=CIRCLE('',#21520,0.01290000000001);
#7724=CIRCLE('',#21521,0.01290000000001);
#7725=CIRCLE('',#21522,0.01290000000001);
#7726=CIRCLE('',#21523,0.01290000000001);
#7727=CIRCLE('',#21524,0.01290000000001);
#7728=CIRCLE('',#21525,0.01290000000001);
#7729=CIRCLE('',#21526,0.01290000000001);
#7730=CIRCLE('',#21527,0.01290000000001);
#7731=CIRCLE('',#21528,0.01290000000001);
#7732=CIRCLE('',#21529,0.01290000000001);
#7733=CIRCLE('',#21530,0.01290000000001);
#7734=CIRCLE('',#21531,0.01290000000001);
#7735=CIRCLE('',#21532,0.01290000000001);
#7736=CIRCLE('',#21533,0.01290000000001);
#7737=CIRCLE('',#21534,0.01290000000001);
#7738=CIRCLE('',#21535,0.01290000000001);
#7739=CIRCLE('',#21536,0.01290000000001);
#7740=CIRCLE('',#21537,0.01290000000001);
#7741=CIRCLE('',#21538,0.01290000000001);
#7742=CIRCLE('',#21539,0.01290000000001);
#7743=CIRCLE('',#21540,0.01290000000001);
#7744=CIRCLE('',#21541,0.01290000000001);
#7745=CIRCLE('',#21542,0.01290000000001);
#7746=CIRCLE('',#21543,0.01290000000001);
#7747=CIRCLE('',#21544,0.01290000000001);
#7748=CIRCLE('',#21545,0.01290000000001);
#7749=CIRCLE('',#21546,0.01290000000001);
#7750=CIRCLE('',#21547,0.01290000000001);
#7751=CIRCLE('',#21548,0.01290000000001);
#7752=CIRCLE('',#21549,0.01290000000001);
#7753=CIRCLE('',#21550,0.01290000000001);
#7754=CIRCLE('',#21551,0.01290000000001);
#7755=CIRCLE('',#21552,0.01290000000001);
#7756=CIRCLE('',#21553,0.01290000000001);
#7757=CIRCLE('',#21554,0.00250000000001);
#7758=CIRCLE('',#21556,0.01290000000001);
#7759=CIRCLE('',#21558,0.01290000000001);
#7760=CIRCLE('',#21560,0.01290000000001);
#7761=CIRCLE('',#21562,0.01290000000001);
#7762=CIRCLE('',#21564,0.01290000000001);
#7763=CIRCLE('',#21566,0.01290000000001);
#7764=CIRCLE('',#21568,0.01290000000001);
#7765=CIRCLE('',#21570,0.01290000000001);
#7766=CIRCLE('',#21572,0.01290000000001);
#7767=CIRCLE('',#21574,0.01290000000001);
#7768=CIRCLE('',#21576,0.01290000000001);
#7769=CIRCLE('',#21578,0.01290000000001);
#7770=CIRCLE('',#21580,0.01290000000001);
#7771=CIRCLE('',#21582,0.01290000000001);
#7772=CIRCLE('',#21584,0.01290000000001);
#7773=CIRCLE('',#21586,0.01290000000001);
#7774=CIRCLE('',#21588,0.01290000000001);
#7775=CIRCLE('',#21590,0.01290000000001);
#7776=CIRCLE('',#21592,0.01290000000001);
#7777=CIRCLE('',#21594,0.01290000000001);
#7778=CIRCLE('',#21596,0.01290000000001);
#7779=CIRCLE('',#21598,0.01290000000001);
#7780=CIRCLE('',#21600,0.01290000000001);
#7781=CIRCLE('',#21602,0.01290000000001);
#7782=CIRCLE('',#21604,0.01290000000001);
#7783=CIRCLE('',#21606,0.01290000000001);
#7784=CIRCLE('',#21608,0.01290000000001);
#7785=CIRCLE('',#21610,0.01290000000001);
#7786=CIRCLE('',#21612,0.01290000000001);
#7787=CIRCLE('',#21614,0.01290000000001);
#7788=CIRCLE('',#21616,0.01290000000001);
#7789=CIRCLE('',#21618,0.01290000000001);
#7790=CIRCLE('',#21620,0.01290000000001);
#7791=CIRCLE('',#21622,0.01290000000001);
#7792=CIRCLE('',#21624,0.01290000000001);
#7793=CIRCLE('',#21626,0.01290000000001);
#7794=CIRCLE('',#21628,0.01290000000001);
#7795=CIRCLE('',#21630,0.01290000000001);
#7796=CIRCLE('',#21632,0.01290000000001);
#7797=CIRCLE('',#21634,0.01290000000001);
#7798=CIRCLE('',#21636,0.01290000000001);
#7799=CIRCLE('',#21638,0.01290000000001);
#7800=CIRCLE('',#21640,0.01290000000001);
#7801=CIRCLE('',#21642,0.01290000000001);
#7802=CIRCLE('',#21644,0.00050000000001);
#7803=CIRCLE('',#21646,0.01290000000001);
#7804=CIRCLE('',#21647,0.00250000000001);
#9241=VERTEX_POINT('',#32382);
#9242=VERTEX_POINT('',#32383);
#9243=VERTEX_POINT('',#32385);
#9244=VERTEX_POINT('',#32387);
#9245=VERTEX_POINT('',#32391);
#9246=VERTEX_POINT('',#32392);
#9247=VERTEX_POINT('',#32394);
#9248=VERTEX_POINT('',#32396);
#9249=VERTEX_POINT('',#32400);
#9250=VERTEX_POINT('',#32401);
#9251=VERTEX_POINT('',#32403);
#9252=VERTEX_POINT('',#32405);
#9253=VERTEX_POINT('',#32409);
#9254=VERTEX_POINT('',#32410);
#9255=VERTEX_POINT('',#32412);
#9256=VERTEX_POINT('',#32414);
#9257=VERTEX_POINT('',#32418);
#9258=VERTEX_POINT('',#32419);
#9259=VERTEX_POINT('',#32421);
#9260=VERTEX_POINT('',#32423);
#9261=VERTEX_POINT('',#32427);
#9262=VERTEX_POINT('',#32428);
#9263=VERTEX_POINT('',#32430);
#9264=VERTEX_POINT('',#32432);
#9265=VERTEX_POINT('',#32436);
#9266=VERTEX_POINT('',#32437);
#9267=VERTEX_POINT('',#32439);
#9268=VERTEX_POINT('',#32441);
#9269=VERTEX_POINT('',#32445);
#9270=VERTEX_POINT('',#32446);
#9271=VERTEX_POINT('',#32448);
#9272=VERTEX_POINT('',#32450);
#9273=VERTEX_POINT('',#32454);
#9274=VERTEX_POINT('',#32455);
#9275=VERTEX_POINT('',#32457);
#9276=VERTEX_POINT('',#32459);
#9277=VERTEX_POINT('',#32463);
#9278=VERTEX_POINT('',#32464);
#9279=VERTEX_POINT('',#32466);
#9280=VERTEX_POINT('',#32468);
#9281=VERTEX_POINT('',#32472);
#9282=VERTEX_POINT('',#32473);
#9283=VERTEX_POINT('',#32475);
#9284=VERTEX_POINT('',#32477);
#9285=VERTEX_POINT('',#32481);
#9286=VERTEX_POINT('',#32482);
#9287=VERTEX_POINT('',#32484);
#9288=VERTEX_POINT('',#32486);
#9289=VERTEX_POINT('',#32490);
#9290=VERTEX_POINT('',#32491);
#9291=VERTEX_POINT('',#32493);
#9292=VERTEX_POINT('',#32495);
#9293=VERTEX_POINT('',#32499);
#9294=VERTEX_POINT('',#32500);
#9295=VERTEX_POINT('',#32502);
#9296=VERTEX_POINT('',#32504);
#9297=VERTEX_POINT('',#32508);
#9298=VERTEX_POINT('',#32509);
#9299=VERTEX_POINT('',#32511);
#9300=VERTEX_POINT('',#32513);
#9301=VERTEX_POINT('',#32517);
#9302=VERTEX_POINT('',#32518);
#9303=VERTEX_POINT('',#32520);
#9304=VERTEX_POINT('',#32522);
#9305=VERTEX_POINT('',#32526);
#9306=VERTEX_POINT('',#32527);
#9307=VERTEX_POINT('',#32529);
#9308=VERTEX_POINT('',#32531);
#9309=VERTEX_POINT('',#32535);
#9310=VERTEX_POINT('',#32536);
#9311=VERTEX_POINT('',#32538);
#9312=VERTEX_POINT('',#32540);
#9313=VERTEX_POINT('',#32544);
#9314=VERTEX_POINT('',#32545);
#9315=VERTEX_POINT('',#32547);
#9316=VERTEX_POINT('',#32549);
#9317=VERTEX_POINT('',#32553);
#9318=VERTEX_POINT('',#32554);
#9319=VERTEX_POINT('',#32556);
#9320=VERTEX_POINT('',#32558);
#9321=VERTEX_POINT('',#32562);
#9322=VERTEX_POINT('',#32563);
#9323=VERTEX_POINT('',#32565);
#9324=VERTEX_POINT('',#32567);
#9325=VERTEX_POINT('',#32571);
#9326=VERTEX_POINT('',#32572);
#9327=VERTEX_POINT('',#32574);
#9328=VERTEX_POINT('',#32576);
#9329=VERTEX_POINT('',#32580);
#9330=VERTEX_POINT('',#32581);
#9331=VERTEX_POINT('',#32583);
#9332=VERTEX_POINT('',#32585);
#9333=VERTEX_POINT('',#32589);
#9334=VERTEX_POINT('',#32590);
#9335=VERTEX_POINT('',#32592);
#9336=VERTEX_POINT('',#32594);
#9337=VERTEX_POINT('',#32598);
#9338=VERTEX_POINT('',#32599);
#9339=VERTEX_POINT('',#32601);
#9340=VERTEX_POINT('',#32603);
#9341=VERTEX_POINT('',#32607);
#9342=VERTEX_POINT('',#32608);
#9343=VERTEX_POINT('',#32610);
#9344=VERTEX_POINT('',#32612);
#9345=VERTEX_POINT('',#32616);
#9346=VERTEX_POINT('',#32617);
#9347=VERTEX_POINT('',#32619);
#9348=VERTEX_POINT('',#32621);
#9349=VERTEX_POINT('',#32625);
#9350=VERTEX_POINT('',#32626);
#9351=VERTEX_POINT('',#32628);
#9352=VERTEX_POINT('',#32630);
#9353=VERTEX_POINT('',#32634);
#9354=VERTEX_POINT('',#32635);
#9355=VERTEX_POINT('',#32637);
#9356=VERTEX_POINT('',#32639);
#9357=VERTEX_POINT('',#32643);
#9358=VERTEX_POINT('',#32644);
#9359=VERTEX_POINT('',#32646);
#9360=VERTEX_POINT('',#32648);
#9361=VERTEX_POINT('',#32652);
#9362=VERTEX_POINT('',#32653);
#9363=VERTEX_POINT('',#32655);
#9364=VERTEX_POINT('',#32657);
#9365=VERTEX_POINT('',#32661);
#9366=VERTEX_POINT('',#32662);
#9367=VERTEX_POINT('',#32664);
#9368=VERTEX_POINT('',#32666);
#9369=VERTEX_POINT('',#32670);
#9370=VERTEX_POINT('',#32671);
#9371=VERTEX_POINT('',#32673);
#9372=VERTEX_POINT('',#32675);
#9373=VERTEX_POINT('',#32679);
#9374=VERTEX_POINT('',#32680);
#9375=VERTEX_POINT('',#32682);
#9376=VERTEX_POINT('',#32684);
#9377=VERTEX_POINT('',#32688);
#9378=VERTEX_POINT('',#32689);
#9379=VERTEX_POINT('',#32691);
#9380=VERTEX_POINT('',#32693);
#9381=VERTEX_POINT('',#32697);
#9382=VERTEX_POINT('',#32698);
#9383=VERTEX_POINT('',#32700);
#9384=VERTEX_POINT('',#32702);
#9385=VERTEX_POINT('',#32706);
#9386=VERTEX_POINT('',#32707);
#9387=VERTEX_POINT('',#32709);
#9388=VERTEX_POINT('',#32711);
#9389=VERTEX_POINT('',#32715);
#9390=VERTEX_POINT('',#32716);
#9391=VERTEX_POINT('',#32718);
#9392=VERTEX_POINT('',#32720);
#9393=VERTEX_POINT('',#32724);
#9394=VERTEX_POINT('',#32725);
#9395=VERTEX_POINT('',#32727);
#9396=VERTEX_POINT('',#32729);
#9397=VERTEX_POINT('',#32733);
#9398=VERTEX_POINT('',#32734);
#9399=VERTEX_POINT('',#32736);
#9400=VERTEX_POINT('',#32738);
#9401=VERTEX_POINT('',#32742);
#9402=VERTEX_POINT('',#32743);
#9403=VERTEX_POINT('',#32745);
#9404=VERTEX_POINT('',#32747);
#9405=VERTEX_POINT('',#32751);
#9406=VERTEX_POINT('',#32752);
#9407=VERTEX_POINT('',#32754);
#9408=VERTEX_POINT('',#32756);
#9409=VERTEX_POINT('',#32760);
#9410=VERTEX_POINT('',#32761);
#9411=VERTEX_POINT('',#32763);
#9412=VERTEX_POINT('',#32765);
#9413=VERTEX_POINT('',#32769);
#9414=VERTEX_POINT('',#32770);
#9415=VERTEX_POINT('',#32772);
#9416=VERTEX_POINT('',#32774);
#9417=VERTEX_POINT('',#32778);
#9418=VERTEX_POINT('',#32780);
#9419=VERTEX_POINT('',#32826);
#9420=VERTEX_POINT('',#32829);
#9421=VERTEX_POINT('',#32833);
#9422=VERTEX_POINT('',#32924);
#11725=EDGE_CURVE('',#9241,#9242,#2083,.T.);
#11726=EDGE_CURVE('',#9243,#9241,#7623,.T.);
#11727=EDGE_CURVE('',#9244,#9243,#2084,.T.);
#11728=EDGE_CURVE('',#9242,#9244,#7624,.T.);
#11729=EDGE_CURVE('',#9245,#9246,#2085,.T.);
#11730=EDGE_CURVE('',#9247,#9245,#7625,.T.);
#11731=EDGE_CURVE('',#9248,#9247,#2086,.T.);
#11732=EDGE_CURVE('',#9246,#9248,#7626,.T.);
#11733=EDGE_CURVE('',#9249,#9250,#2087,.T.);
#11734=EDGE_CURVE('',#9251,#9249,#7627,.T.);
#11735=EDGE_CURVE('',#9252,#9251,#2088,.T.);
#11736=EDGE_CURVE('',#9250,#9252,#7628,.T.);
#11737=EDGE_CURVE('',#9253,#9254,#2089,.T.);
#11738=EDGE_CURVE('',#9255,#9253,#7629,.T.);
#11739=EDGE_CURVE('',#9256,#9255,#2090,.T.);
#11740=EDGE_CURVE('',#9254,#9256,#7630,.T.);
#11741=EDGE_CURVE('',#9257,#9258,#2091,.T.);
#11742=EDGE_CURVE('',#9259,#9257,#7631,.T.);
#11743=EDGE_CURVE('',#9260,#9259,#2092,.T.);
#11744=EDGE_CURVE('',#9258,#9260,#7632,.T.);
#11745=EDGE_CURVE('',#9261,#9262,#2093,.T.);
#11746=EDGE_CURVE('',#9263,#9261,#7633,.T.);
#11747=EDGE_CURVE('',#9264,#9263,#2094,.T.);
#11748=EDGE_CURVE('',#9262,#9264,#7634,.T.);
#11749=EDGE_CURVE('',#9265,#9266,#2095,.T.);
#11750=EDGE_CURVE('',#9267,#9265,#7635,.T.);
#11751=EDGE_CURVE('',#9268,#9267,#2096,.T.);
#11752=EDGE_CURVE('',#9266,#9268,#7636,.T.);
#11753=EDGE_CURVE('',#9269,#9270,#2097,.T.);
#11754=EDGE_CURVE('',#9271,#9269,#7637,.T.);
#11755=EDGE_CURVE('',#9272,#9271,#2098,.T.);
#11756=EDGE_CURVE('',#9270,#9272,#7638,.T.);
#11757=EDGE_CURVE('',#9273,#9274,#2099,.T.);
#11758=EDGE_CURVE('',#9275,#9273,#7639,.T.);
#11759=EDGE_CURVE('',#9276,#9275,#2100,.T.);
#11760=EDGE_CURVE('',#9274,#9276,#7640,.T.);
#11761=EDGE_CURVE('',#9277,#9278,#2101,.T.);
#11762=EDGE_CURVE('',#9279,#9277,#7641,.T.);
#11763=EDGE_CURVE('',#9280,#9279,#2102,.T.);
#11764=EDGE_CURVE('',#9278,#9280,#7642,.T.);
#11765=EDGE_CURVE('',#9281,#9282,#2103,.T.);
#11766=EDGE_CURVE('',#9283,#9281,#7643,.T.);
#11767=EDGE_CURVE('',#9284,#9283,#2104,.T.);
#11768=EDGE_CURVE('',#9282,#9284,#7644,.T.);
#11769=EDGE_CURVE('',#9285,#9286,#2105,.T.);
#11770=EDGE_CURVE('',#9287,#9285,#7645,.T.);
#11771=EDGE_CURVE('',#9288,#9287,#2106,.T.);
#11772=EDGE_CURVE('',#9286,#9288,#7646,.T.);
#11773=EDGE_CURVE('',#9289,#9290,#2107,.T.);
#11774=EDGE_CURVE('',#9291,#9289,#7647,.T.);
#11775=EDGE_CURVE('',#9292,#9291,#2108,.T.);
#11776=EDGE_CURVE('',#9290,#9292,#7648,.T.);
#11777=EDGE_CURVE('',#9293,#9294,#2109,.T.);
#11778=EDGE_CURVE('',#9295,#9293,#7649,.T.);
#11779=EDGE_CURVE('',#9296,#9295,#2110,.T.);
#11780=EDGE_CURVE('',#9294,#9296,#7650,.T.);
#11781=EDGE_CURVE('',#9297,#9298,#2111,.T.);
#11782=EDGE_CURVE('',#9299,#9297,#7651,.T.);
#11783=EDGE_CURVE('',#9300,#9299,#2112,.T.);
#11784=EDGE_CURVE('',#9298,#9300,#7652,.T.);
#11785=EDGE_CURVE('',#9301,#9302,#2113,.T.);
#11786=EDGE_CURVE('',#9303,#9301,#7653,.T.);
#11787=EDGE_CURVE('',#9304,#9303,#2114,.T.);
#11788=EDGE_CURVE('',#9302,#9304,#7654,.T.);
#11789=EDGE_CURVE('',#9305,#9306,#2115,.T.);
#11790=EDGE_CURVE('',#9307,#9305,#7655,.T.);
#11791=EDGE_CURVE('',#9308,#9307,#2116,.T.);
#11792=EDGE_CURVE('',#9306,#9308,#7656,.T.);
#11793=EDGE_CURVE('',#9309,#9310,#2117,.T.);
#11794=EDGE_CURVE('',#9311,#9309,#7657,.T.);
#11795=EDGE_CURVE('',#9312,#9311,#2118,.T.);
#11796=EDGE_CURVE('',#9310,#9312,#7658,.T.);
#11797=EDGE_CURVE('',#9313,#9314,#2119,.T.);
#11798=EDGE_CURVE('',#9315,#9313,#7659,.T.);
#11799=EDGE_CURVE('',#9316,#9315,#2120,.T.);
#11800=EDGE_CURVE('',#9314,#9316,#7660,.T.);
#11801=EDGE_CURVE('',#9317,#9318,#2121,.T.);
#11802=EDGE_CURVE('',#9319,#9317,#7661,.T.);
#11803=EDGE_CURVE('',#9320,#9319,#2122,.T.);
#11804=EDGE_CURVE('',#9318,#9320,#7662,.T.);
#11805=EDGE_CURVE('',#9321,#9322,#2123,.T.);
#11806=EDGE_CURVE('',#9323,#9321,#7663,.T.);
#11807=EDGE_CURVE('',#9324,#9323,#2124,.T.);
#11808=EDGE_CURVE('',#9322,#9324,#7664,.T.);
#11809=EDGE_CURVE('',#9325,#9326,#2125,.T.);
#11810=EDGE_CURVE('',#9327,#9325,#7665,.T.);
#11811=EDGE_CURVE('',#9328,#9327,#2126,.T.);
#11812=EDGE_CURVE('',#9326,#9328,#7666,.T.);
#11813=EDGE_CURVE('',#9329,#9330,#2127,.T.);
#11814=EDGE_CURVE('',#9331,#9329,#7667,.T.);
#11815=EDGE_CURVE('',#9332,#9331,#2128,.T.);
#11816=EDGE_CURVE('',#9330,#9332,#7668,.T.);
#11817=EDGE_CURVE('',#9333,#9334,#2129,.T.);
#11818=EDGE_CURVE('',#9335,#9333,#7669,.T.);
#11819=EDGE_CURVE('',#9336,#9335,#2130,.T.);
#11820=EDGE_CURVE('',#9334,#9336,#7670,.T.);
#11821=EDGE_CURVE('',#9337,#9338,#2131,.T.);
#11822=EDGE_CURVE('',#9339,#9337,#7671,.T.);
#11823=EDGE_CURVE('',#9340,#9339,#2132,.T.);
#11824=EDGE_CURVE('',#9338,#9340,#7672,.T.);
#11825=EDGE_CURVE('',#9341,#9342,#2133,.T.);
#11826=EDGE_CURVE('',#9343,#9341,#7673,.T.);
#11827=EDGE_CURVE('',#9344,#9343,#2134,.T.);
#11828=EDGE_CURVE('',#9342,#9344,#7674,.T.);
#11829=EDGE_CURVE('',#9345,#9346,#2135,.T.);
#11830=EDGE_CURVE('',#9347,#9345,#7675,.T.);
#11831=EDGE_CURVE('',#9348,#9347,#2136,.T.);
#11832=EDGE_CURVE('',#9346,#9348,#7676,.T.);
#11833=EDGE_CURVE('',#9349,#9350,#2137,.T.);
#11834=EDGE_CURVE('',#9351,#9349,#7677,.T.);
#11835=EDGE_CURVE('',#9352,#9351,#2138,.T.);
#11836=EDGE_CURVE('',#9350,#9352,#7678,.T.);
#11837=EDGE_CURVE('',#9353,#9354,#2139,.T.);
#11838=EDGE_CURVE('',#9355,#9353,#7679,.T.);
#11839=EDGE_CURVE('',#9356,#9355,#2140,.T.);
#11840=EDGE_CURVE('',#9354,#9356,#7680,.T.);
#11841=EDGE_CURVE('',#9357,#9358,#2141,.T.);
#11842=EDGE_CURVE('',#9359,#9357,#7681,.T.);
#11843=EDGE_CURVE('',#9360,#9359,#2142,.T.);
#11844=EDGE_CURVE('',#9358,#9360,#7682,.T.);
#11845=EDGE_CURVE('',#9361,#9362,#2143,.T.);
#11846=EDGE_CURVE('',#9363,#9361,#7683,.T.);
#11847=EDGE_CURVE('',#9364,#9363,#2144,.T.);
#11848=EDGE_CURVE('',#9362,#9364,#7684,.T.);
#11849=EDGE_CURVE('',#9365,#9366,#2145,.T.);
#11850=EDGE_CURVE('',#9367,#9365,#7685,.T.);
#11851=EDGE_CURVE('',#9368,#9367,#2146,.T.);
#11852=EDGE_CURVE('',#9366,#9368,#7686,.T.);
#11853=EDGE_CURVE('',#9369,#9370,#2147,.T.);
#11854=EDGE_CURVE('',#9371,#9369,#7687,.T.);
#11855=EDGE_CURVE('',#9372,#9371,#2148,.T.);
#11856=EDGE_CURVE('',#9370,#9372,#7688,.T.);
#11857=EDGE_CURVE('',#9373,#9374,#2149,.T.);
#11858=EDGE_CURVE('',#9375,#9373,#7689,.T.);
#11859=EDGE_CURVE('',#9376,#9375,#2150,.T.);
#11860=EDGE_CURVE('',#9374,#9376,#7690,.T.);
#11861=EDGE_CURVE('',#9377,#9378,#2151,.T.);
#11862=EDGE_CURVE('',#9379,#9377,#7691,.T.);
#11863=EDGE_CURVE('',#9380,#9379,#2152,.T.);
#11864=EDGE_CURVE('',#9378,#9380,#7692,.T.);
#11865=EDGE_CURVE('',#9381,#9382,#2153,.T.);
#11866=EDGE_CURVE('',#9383,#9381,#7693,.T.);
#11867=EDGE_CURVE('',#9384,#9383,#2154,.T.);
#11868=EDGE_CURVE('',#9382,#9384,#7694,.T.);
#11869=EDGE_CURVE('',#9385,#9386,#2155,.T.);
#11870=EDGE_CURVE('',#9387,#9385,#7695,.T.);
#11871=EDGE_CURVE('',#9388,#9387,#2156,.T.);
#11872=EDGE_CURVE('',#9386,#9388,#7696,.T.);
#11873=EDGE_CURVE('',#9389,#9390,#2157,.T.);
#11874=EDGE_CURVE('',#9391,#9389,#7697,.T.);
#11875=EDGE_CURVE('',#9392,#9391,#2158,.T.);
#11876=EDGE_CURVE('',#9390,#9392,#7698,.T.);
#11877=EDGE_CURVE('',#9393,#9394,#2159,.T.);
#11878=EDGE_CURVE('',#9395,#9393,#7699,.T.);
#11879=EDGE_CURVE('',#9396,#9395,#2160,.T.);
#11880=EDGE_CURVE('',#9394,#9396,#7700,.T.);
#11881=EDGE_CURVE('',#9397,#9398,#2161,.T.);
#11882=EDGE_CURVE('',#9399,#9397,#7701,.T.);
#11883=EDGE_CURVE('',#9400,#9399,#2162,.T.);
#11884=EDGE_CURVE('',#9398,#9400,#7702,.T.);
#11885=EDGE_CURVE('',#9401,#9402,#2163,.T.);
#11886=EDGE_CURVE('',#9403,#9401,#7703,.T.);
#11887=EDGE_CURVE('',#9404,#9403,#2164,.T.);
#11888=EDGE_CURVE('',#9402,#9404,#7704,.T.);
#11889=EDGE_CURVE('',#9405,#9406,#2165,.T.);
#11890=EDGE_CURVE('',#9407,#9405,#7705,.T.);
#11891=EDGE_CURVE('',#9408,#9407,#2166,.T.);
#11892=EDGE_CURVE('',#9406,#9408,#7706,.T.);
#11893=EDGE_CURVE('',#9409,#9410,#2167,.T.);
#11894=EDGE_CURVE('',#9411,#9409,#7707,.T.);
#11895=EDGE_CURVE('',#9412,#9411,#2168,.T.);
#11896=EDGE_CURVE('',#9410,#9412,#7708,.T.);
#11897=EDGE_CURVE('',#9413,#9414,#2169,.T.);
#11898=EDGE_CURVE('',#9415,#9413,#7709,.T.);
#11899=EDGE_CURVE('',#9416,#9415,#2170,.T.);
#11900=EDGE_CURVE('',#9414,#9416,#7710,.T.);
#11901=EDGE_CURVE('',#9241,#9417,#7711,.T.);
#11902=EDGE_CURVE('',#9417,#9418,#7712,.T.);
#11903=EDGE_CURVE('',#9418,#9415,#7713,.T.);
#11904=EDGE_CURVE('',#9413,#9411,#7714,.T.);
#11905=EDGE_CURVE('',#9409,#9407,#7715,.T.);
#11906=EDGE_CURVE('',#9405,#9403,#7716,.T.);
#11907=EDGE_CURVE('',#9401,#9399,#7717,.T.);
#11908=EDGE_CURVE('',#9397,#9395,#7718,.T.);
#11909=EDGE_CURVE('',#9393,#9391,#7719,.T.);
#11910=EDGE_CURVE('',#9389,#9387,#7720,.T.);
#11911=EDGE_CURVE('',#9385,#9383,#7721,.T.);
#11912=EDGE_CURVE('',#9381,#9379,#7722,.T.);
#11913=EDGE_CURVE('',#9377,#9375,#7723,.T.);
#11914=EDGE_CURVE('',#9373,#9371,#7724,.T.);
#11915=EDGE_CURVE('',#9369,#9367,#7725,.T.);
#11916=EDGE_CURVE('',#9365,#9363,#7726,.T.);
#11917=EDGE_CURVE('',#9361,#9359,#7727,.T.);
#11918=EDGE_CURVE('',#9357,#9355,#7728,.T.);
#11919=EDGE_CURVE('',#9353,#9351,#7729,.T.);
#11920=EDGE_CURVE('',#9349,#9347,#7730,.T.);
#11921=EDGE_CURVE('',#9345,#9343,#7731,.T.);
#11922=EDGE_CURVE('',#9341,#9339,#7732,.T.);
#11923=EDGE_CURVE('',#9337,#9335,#7733,.T.);
#11924=EDGE_CURVE('',#9333,#9331,#7734,.T.);
#11925=EDGE_CURVE('',#9329,#9327,#7735,.T.);
#11926=EDGE_CURVE('',#9325,#9323,#7736,.T.);
#11927=EDGE_CURVE('',#9321,#9319,#7737,.T.);
#11928=EDGE_CURVE('',#9317,#9315,#7738,.T.);
#11929=EDGE_CURVE('',#9313,#9311,#7739,.T.);
#11930=EDGE_CURVE('',#9309,#9307,#7740,.T.);
#11931=EDGE_CURVE('',#9305,#9303,#7741,.T.);
#11932=EDGE_CURVE('',#9301,#9299,#7742,.T.);
#11933=EDGE_CURVE('',#9297,#9295,#7743,.T.);
#11934=EDGE_CURVE('',#9293,#9291,#7744,.T.);
#11935=EDGE_CURVE('',#9289,#9287,#7745,.T.);
#11936=EDGE_CURVE('',#9285,#9283,#7746,.T.);
#11937=EDGE_CURVE('',#9281,#9279,#7747,.T.);
#11938=EDGE_CURVE('',#9277,#9275,#7748,.T.);
#11939=EDGE_CURVE('',#9273,#9271,#7749,.T.);
#11940=EDGE_CURVE('',#9269,#9267,#7750,.T.);
#11941=EDGE_CURVE('',#9265,#9263,#7751,.T.);
#11942=EDGE_CURVE('',#9261,#9259,#7752,.T.);
#11943=EDGE_CURVE('',#9257,#9255,#7753,.T.);
#11944=EDGE_CURVE('',#9253,#9251,#7754,.T.);
#11945=EDGE_CURVE('',#9249,#9247,#7755,.T.);
#11946=EDGE_CURVE('',#9245,#9243,#7756,.T.);
#11947=EDGE_CURVE('',#9419,#9419,#7757,.T.);
#11948=EDGE_CURVE('',#9242,#9420,#7758,.T.);
#11949=EDGE_CURVE('',#9420,#9417,#2171,.T.);
#11950=EDGE_CURVE('',#9418,#9421,#2172,.T.);
#11951=EDGE_CURVE('',#9421,#9416,#7759,.T.);
#11952=EDGE_CURVE('',#9414,#9412,#7760,.T.);
#11953=EDGE_CURVE('',#9410,#9408,#7761,.T.);
#11954=EDGE_CURVE('',#9406,#9404,#7762,.T.);
#11955=EDGE_CURVE('',#9402,#9400,#7763,.T.);
#11956=EDGE_CURVE('',#9398,#9396,#7764,.T.);
#11957=EDGE_CURVE('',#9394,#9392,#7765,.T.);
#11958=EDGE_CURVE('',#9390,#9388,#7766,.T.);
#11959=EDGE_CURVE('',#9386,#9384,#7767,.T.);
#11960=EDGE_CURVE('',#9382,#9380,#7768,.T.);
#11961=EDGE_CURVE('',#9378,#9376,#7769,.T.);
#11962=EDGE_CURVE('',#9374,#9372,#7770,.T.);
#11963=EDGE_CURVE('',#9370,#9368,#7771,.T.);
#11964=EDGE_CURVE('',#9366,#9364,#7772,.T.);
#11965=EDGE_CURVE('',#9362,#9360,#7773,.T.);
#11966=EDGE_CURVE('',#9358,#9356,#7774,.T.);
#11967=EDGE_CURVE('',#9354,#9352,#7775,.T.);
#11968=EDGE_CURVE('',#9350,#9348,#7776,.T.);
#11969=EDGE_CURVE('',#9346,#9344,#7777,.T.);
#11970=EDGE_CURVE('',#9342,#9340,#7778,.T.);
#11971=EDGE_CURVE('',#9338,#9336,#7779,.T.);
#11972=EDGE_CURVE('',#9334,#9332,#7780,.T.);
#11973=EDGE_CURVE('',#9330,#9328,#7781,.T.);
#11974=EDGE_CURVE('',#9326,#9324,#7782,.T.);
#11975=EDGE_CURVE('',#9322,#9320,#7783,.T.);
#11976=EDGE_CURVE('',#9318,#9316,#7784,.T.);
#11977=EDGE_CURVE('',#9314,#9312,#7785,.T.);
#11978=EDGE_CURVE('',#9310,#9308,#7786,.T.);
#11979=EDGE_CURVE('',#9306,#9304,#7787,.T.);
#11980=EDGE_CURVE('',#9302,#9300,#7788,.T.);
#11981=EDGE_CURVE('',#9298,#9296,#7789,.T.);
#11982=EDGE_CURVE('',#9294,#9292,#7790,.T.);
#11983=EDGE_CURVE('',#9290,#9288,#7791,.T.);
#11984=EDGE_CURVE('',#9286,#9284,#7792,.T.);
#11985=EDGE_CURVE('',#9282,#9280,#7793,.T.);
#11986=EDGE_CURVE('',#9278,#9276,#7794,.T.);
#11987=EDGE_CURVE('',#9274,#9272,#7795,.T.);
#11988=EDGE_CURVE('',#9270,#9268,#7796,.T.);
#11989=EDGE_CURVE('',#9266,#9264,#7797,.T.);
#11990=EDGE_CURVE('',#9262,#9260,#7798,.T.);
#11991=EDGE_CURVE('',#9258,#9256,#7799,.T.);
#11992=EDGE_CURVE('',#9254,#9252,#7800,.T.);
#11993=EDGE_CURVE('',#9250,#9248,#7801,.T.);
#11994=EDGE_CURVE('',#9421,#9420,#7802,.T.);
#11995=EDGE_CURVE('',#9246,#9244,#7803,.T.);
#11996=EDGE_CURVE('',#9422,#9422,#7804,.T.);
#11997=EDGE_CURVE('',#9422,#9419,#2173,.T.);
#16334=ORIENTED_EDGE('',*,*,#11725,.F.);
#16335=ORIENTED_EDGE('',*,*,#11726,.F.);
#16336=ORIENTED_EDGE('',*,*,#11727,.F.);
#16337=ORIENTED_EDGE('',*,*,#11728,.F.);
#16338=ORIENTED_EDGE('',*,*,#11729,.F.);
#16339=ORIENTED_EDGE('',*,*,#11730,.F.);
#16340=ORIENTED_EDGE('',*,*,#11731,.F.);
#16341=ORIENTED_EDGE('',*,*,#11732,.F.);
#16342=ORIENTED_EDGE('',*,*,#11733,.F.);
#16343=ORIENTED_EDGE('',*,*,#11734,.F.);
#16344=ORIENTED_EDGE('',*,*,#11735,.F.);
#16345=ORIENTED_EDGE('',*,*,#11736,.F.);
#16346=ORIENTED_EDGE('',*,*,#11737,.F.);
#16347=ORIENTED_EDGE('',*,*,#11738,.F.);
#16348=ORIENTED_EDGE('',*,*,#11739,.F.);
#16349=ORIENTED_EDGE('',*,*,#11740,.F.);
#16350=ORIENTED_EDGE('',*,*,#11741,.F.);
#16351=ORIENTED_EDGE('',*,*,#11742,.F.);
#16352=ORIENTED_EDGE('',*,*,#11743,.F.);
#16353=ORIENTED_EDGE('',*,*,#11744,.F.);
#16354=ORIENTED_EDGE('',*,*,#11745,.F.);
#16355=ORIENTED_EDGE('',*,*,#11746,.F.);
#16356=ORIENTED_EDGE('',*,*,#11747,.F.);
#16357=ORIENTED_EDGE('',*,*,#11748,.F.);
#16358=ORIENTED_EDGE('',*,*,#11749,.F.);
#16359=ORIENTED_EDGE('',*,*,#11750,.F.);
#16360=ORIENTED_EDGE('',*,*,#11751,.F.);
#16361=ORIENTED_EDGE('',*,*,#11752,.F.);
#16362=ORIENTED_EDGE('',*,*,#11753,.F.);
#16363=ORIENTED_EDGE('',*,*,#11754,.F.);
#16364=ORIENTED_EDGE('',*,*,#11755,.F.);
#16365=ORIENTED_EDGE('',*,*,#11756,.F.);
#16366=ORIENTED_EDGE('',*,*,#11757,.F.);
#16367=ORIENTED_EDGE('',*,*,#11758,.F.);
#16368=ORIENTED_EDGE('',*,*,#11759,.F.);
#16369=ORIENTED_EDGE('',*,*,#11760,.F.);
#16370=ORIENTED_EDGE('',*,*,#11761,.F.);
#16371=ORIENTED_EDGE('',*,*,#11762,.F.);
#16372=ORIENTED_EDGE('',*,*,#11763,.F.);
#16373=ORIENTED_EDGE('',*,*,#11764,.F.);
#16374=ORIENTED_EDGE('',*,*,#11765,.F.);
#16375=ORIENTED_EDGE('',*,*,#11766,.F.);
#16376=ORIENTED_EDGE('',*,*,#11767,.F.);
#16377=ORIENTED_EDGE('',*,*,#11768,.F.);
#16378=ORIENTED_EDGE('',*,*,#11769,.F.);
#16379=ORIENTED_EDGE('',*,*,#11770,.F.);
#16380=ORIENTED_EDGE('',*,*,#11771,.F.);
#16381=ORIENTED_EDGE('',*,*,#11772,.F.);
#16382=ORIENTED_EDGE('',*,*,#11773,.F.);
#16383=ORIENTED_EDGE('',*,*,#11774,.F.);
#16384=ORIENTED_EDGE('',*,*,#11775,.F.);
#16385=ORIENTED_EDGE('',*,*,#11776,.F.);
#16386=ORIENTED_EDGE('',*,*,#11777,.F.);
#16387=ORIENTED_EDGE('',*,*,#11778,.F.);
#16388=ORIENTED_EDGE('',*,*,#11779,.F.);
#16389=ORIENTED_EDGE('',*,*,#11780,.F.);
#16390=ORIENTED_EDGE('',*,*,#11781,.F.);
#16391=ORIENTED_EDGE('',*,*,#11782,.F.);
#16392=ORIENTED_EDGE('',*,*,#11783,.F.);
#16393=ORIENTED_EDGE('',*,*,#11784,.F.);
#16394=ORIENTED_EDGE('',*,*,#11785,.F.);
#16395=ORIENTED_EDGE('',*,*,#11786,.F.);
#16396=ORIENTED_EDGE('',*,*,#11787,.F.);
#16397=ORIENTED_EDGE('',*,*,#11788,.F.);
#16398=ORIENTED_EDGE('',*,*,#11789,.F.);
#16399=ORIENTED_EDGE('',*,*,#11790,.F.);
#16400=ORIENTED_EDGE('',*,*,#11791,.F.);
#16401=ORIENTED_EDGE('',*,*,#11792,.F.);
#16402=ORIENTED_EDGE('',*,*,#11793,.F.);
#16403=ORIENTED_EDGE('',*,*,#11794,.F.);
#16404=ORIENTED_EDGE('',*,*,#11795,.F.);
#16405=ORIENTED_EDGE('',*,*,#11796,.F.);
#16406=ORIENTED_EDGE('',*,*,#11797,.F.);
#16407=ORIENTED_EDGE('',*,*,#11798,.F.);
#16408=ORIENTED_EDGE('',*,*,#11799,.F.);
#16409=ORIENTED_EDGE('',*,*,#11800,.F.);
#16410=ORIENTED_EDGE('',*,*,#11801,.F.);
#16411=ORIENTED_EDGE('',*,*,#11802,.F.);
#16412=ORIENTED_EDGE('',*,*,#11803,.F.);
#16413=ORIENTED_EDGE('',*,*,#11804,.F.);
#16414=ORIENTED_EDGE('',*,*,#11805,.F.);
#16415=ORIENTED_EDGE('',*,*,#11806,.F.);
#16416=ORIENTED_EDGE('',*,*,#11807,.F.);
#16417=ORIENTED_EDGE('',*,*,#11808,.F.);
#16418=ORIENTED_EDGE('',*,*,#11809,.F.);
#16419=ORIENTED_EDGE('',*,*,#11810,.F.);
#16420=ORIENTED_EDGE('',*,*,#11811,.F.);
#16421=ORIENTED_EDGE('',*,*,#11812,.F.);
#16422=ORIENTED_EDGE('',*,*,#11813,.F.);
#16423=ORIENTED_EDGE('',*,*,#11814,.F.);
#16424=ORIENTED_EDGE('',*,*,#11815,.F.);
#16425=ORIENTED_EDGE('',*,*,#11816,.F.);
#16426=ORIENTED_EDGE('',*,*,#11817,.F.);
#16427=ORIENTED_EDGE('',*,*,#11818,.F.);
#16428=ORIENTED_EDGE('',*,*,#11819,.F.);
#16429=ORIENTED_EDGE('',*,*,#11820,.F.);
#16430=ORIENTED_EDGE('',*,*,#11821,.F.);
#16431=ORIENTED_EDGE('',*,*,#11822,.F.);
#16432=ORIENTED_EDGE('',*,*,#11823,.F.);
#16433=ORIENTED_EDGE('',*,*,#11824,.F.);
#16434=ORIENTED_EDGE('',*,*,#11825,.F.);
#16435=ORIENTED_EDGE('',*,*,#11826,.F.);
#16436=ORIENTED_EDGE('',*,*,#11827,.F.);
#16437=ORIENTED_EDGE('',*,*,#11828,.F.);
#16438=ORIENTED_EDGE('',*,*,#11829,.F.);
#16439=ORIENTED_EDGE('',*,*,#11830,.F.);
#16440=ORIENTED_EDGE('',*,*,#11831,.F.);
#16441=ORIENTED_EDGE('',*,*,#11832,.F.);
#16442=ORIENTED_EDGE('',*,*,#11833,.F.);
#16443=ORIENTED_EDGE('',*,*,#11834,.F.);
#16444=ORIENTED_EDGE('',*,*,#11835,.F.);
#16445=ORIENTED_EDGE('',*,*,#11836,.F.);
#16446=ORIENTED_EDGE('',*,*,#11837,.F.);
#16447=ORIENTED_EDGE('',*,*,#11838,.F.);
#16448=ORIENTED_EDGE('',*,*,#11839,.F.);
#16449=ORIENTED_EDGE('',*,*,#11840,.F.);
#16450=ORIENTED_EDGE('',*,*,#11841,.F.);
#16451=ORIENTED_EDGE('',*,*,#11842,.F.);
#16452=ORIENTED_EDGE('',*,*,#11843,.F.);
#16453=ORIENTED_EDGE('',*,*,#11844,.F.);
#16454=ORIENTED_EDGE('',*,*,#11845,.F.);
#16455=ORIENTED_EDGE('',*,*,#11846,.F.);
#16456=ORIENTED_EDGE('',*,*,#11847,.F.);
#16457=ORIENTED_EDGE('',*,*,#11848,.F.);
#16458=ORIENTED_EDGE('',*,*,#11849,.F.);
#16459=ORIENTED_EDGE('',*,*,#11850,.F.);
#16460=ORIENTED_EDGE('',*,*,#11851,.F.);
#16461=ORIENTED_EDGE('',*,*,#11852,.F.);
#16462=ORIENTED_EDGE('',*,*,#11853,.F.);
#16463=ORIENTED_EDGE('',*,*,#11854,.F.);
#16464=ORIENTED_EDGE('',*,*,#11855,.F.);
#16465=ORIENTED_EDGE('',*,*,#11856,.F.);
#16466=ORIENTED_EDGE('',*,*,#11857,.F.);
#16467=ORIENTED_EDGE('',*,*,#11858,.F.);
#16468=ORIENTED_EDGE('',*,*,#11859,.F.);
#16469=ORIENTED_EDGE('',*,*,#11860,.F.);
#16470=ORIENTED_EDGE('',*,*,#11861,.F.);
#16471=ORIENTED_EDGE('',*,*,#11862,.F.);
#16472=ORIENTED_EDGE('',*,*,#11863,.F.);
#16473=ORIENTED_EDGE('',*,*,#11864,.F.);
#16474=ORIENTED_EDGE('',*,*,#11865,.F.);
#16475=ORIENTED_EDGE('',*,*,#11866,.F.);
#16476=ORIENTED_EDGE('',*,*,#11867,.F.);
#16477=ORIENTED_EDGE('',*,*,#11868,.F.);
#16478=ORIENTED_EDGE('',*,*,#11869,.F.);
#16479=ORIENTED_EDGE('',*,*,#11870,.F.);
#16480=ORIENTED_EDGE('',*,*,#11871,.F.);
#16481=ORIENTED_EDGE('',*,*,#11872,.F.);
#16482=ORIENTED_EDGE('',*,*,#11873,.F.);
#16483=ORIENTED_EDGE('',*,*,#11874,.F.);
#16484=ORIENTED_EDGE('',*,*,#11875,.F.);
#16485=ORIENTED_EDGE('',*,*,#11876,.F.);
#16486=ORIENTED_EDGE('',*,*,#11877,.F.);
#16487=ORIENTED_EDGE('',*,*,#11878,.F.);
#16488=ORIENTED_EDGE('',*,*,#11879,.F.);
#16489=ORIENTED_EDGE('',*,*,#11880,.F.);
#16490=ORIENTED_EDGE('',*,*,#11881,.F.);
#16491=ORIENTED_EDGE('',*,*,#11882,.F.);
#16492=ORIENTED_EDGE('',*,*,#11883,.F.);
#16493=ORIENTED_EDGE('',*,*,#11884,.F.);
#16494=ORIENTED_EDGE('',*,*,#11885,.F.);
#16495=ORIENTED_EDGE('',*,*,#11886,.F.);
#16496=ORIENTED_EDGE('',*,*,#11887,.F.);
#16497=ORIENTED_EDGE('',*,*,#11888,.F.);
#16498=ORIENTED_EDGE('',*,*,#11889,.F.);
#16499=ORIENTED_EDGE('',*,*,#11890,.F.);
#16500=ORIENTED_EDGE('',*,*,#11891,.F.);
#16501=ORIENTED_EDGE('',*,*,#11892,.F.);
#16502=ORIENTED_EDGE('',*,*,#11893,.F.);
#16503=ORIENTED_EDGE('',*,*,#11894,.F.);
#16504=ORIENTED_EDGE('',*,*,#11895,.F.);
#16505=ORIENTED_EDGE('',*,*,#11896,.F.);
#16506=ORIENTED_EDGE('',*,*,#11897,.F.);
#16507=ORIENTED_EDGE('',*,*,#11898,.F.);
#16508=ORIENTED_EDGE('',*,*,#11899,.F.);
#16509=ORIENTED_EDGE('',*,*,#11900,.F.);
#16510=ORIENTED_EDGE('',*,*,#11726,.T.);
#16511=ORIENTED_EDGE('',*,*,#11901,.T.);
#16512=ORIENTED_EDGE('',*,*,#11902,.T.);
#16513=ORIENTED_EDGE('',*,*,#11903,.T.);
#16514=ORIENTED_EDGE('',*,*,#11898,.T.);
#16515=ORIENTED_EDGE('',*,*,#11904,.T.);
#16516=ORIENTED_EDGE('',*,*,#11894,.T.);
#16517=ORIENTED_EDGE('',*,*,#11905,.T.);
#16518=ORIENTED_EDGE('',*,*,#11890,.T.);
#16519=ORIENTED_EDGE('',*,*,#11906,.T.);
#16520=ORIENTED_EDGE('',*,*,#11886,.T.);
#16521=ORIENTED_EDGE('',*,*,#11907,.T.);
#16522=ORIENTED_EDGE('',*,*,#11882,.T.);
#16523=ORIENTED_EDGE('',*,*,#11908,.T.);
#16524=ORIENTED_EDGE('',*,*,#11878,.T.);
#16525=ORIENTED_EDGE('',*,*,#11909,.T.);
#16526=ORIENTED_EDGE('',*,*,#11874,.T.);
#16527=ORIENTED_EDGE('',*,*,#11910,.T.);
#16528=ORIENTED_EDGE('',*,*,#11870,.T.);
#16529=ORIENTED_EDGE('',*,*,#11911,.T.);
#16530=ORIENTED_EDGE('',*,*,#11866,.T.);
#16531=ORIENTED_EDGE('',*,*,#11912,.T.);
#16532=ORIENTED_EDGE('',*,*,#11862,.T.);
#16533=ORIENTED_EDGE('',*,*,#11913,.T.);
#16534=ORIENTED_EDGE('',*,*,#11858,.T.);
#16535=ORIENTED_EDGE('',*,*,#11914,.T.);
#16536=ORIENTED_EDGE('',*,*,#11854,.T.);
#16537=ORIENTED_EDGE('',*,*,#11915,.T.);
#16538=ORIENTED_EDGE('',*,*,#11850,.T.);
#16539=ORIENTED_EDGE('',*,*,#11916,.T.);
#16540=ORIENTED_EDGE('',*,*,#11846,.T.);
#16541=ORIENTED_EDGE('',*,*,#11917,.T.);
#16542=ORIENTED_EDGE('',*,*,#11842,.T.);
#16543=ORIENTED_EDGE('',*,*,#11918,.T.);
#16544=ORIENTED_EDGE('',*,*,#11838,.T.);
#16545=ORIENTED_EDGE('',*,*,#11919,.T.);
#16546=ORIENTED_EDGE('',*,*,#11834,.T.);
#16547=ORIENTED_EDGE('',*,*,#11920,.T.);
#16548=ORIENTED_EDGE('',*,*,#11830,.T.);
#16549=ORIENTED_EDGE('',*,*,#11921,.T.);
#16550=ORIENTED_EDGE('',*,*,#11826,.T.);
#16551=ORIENTED_EDGE('',*,*,#11922,.T.);
#16552=ORIENTED_EDGE('',*,*,#11822,.T.);
#16553=ORIENTED_EDGE('',*,*,#11923,.T.);
#16554=ORIENTED_EDGE('',*,*,#11818,.T.);
#16555=ORIENTED_EDGE('',*,*,#11924,.T.);
#16556=ORIENTED_EDGE('',*,*,#11814,.T.);
#16557=ORIENTED_EDGE('',*,*,#11925,.T.);
#16558=ORIENTED_EDGE('',*,*,#11810,.T.);
#16559=ORIENTED_EDGE('',*,*,#11926,.T.);
#16560=ORIENTED_EDGE('',*,*,#11806,.T.);
#16561=ORIENTED_EDGE('',*,*,#11927,.T.);
#16562=ORIENTED_EDGE('',*,*,#11802,.T.);
#16563=ORIENTED_EDGE('',*,*,#11928,.T.);
#16564=ORIENTED_EDGE('',*,*,#11798,.T.);
#16565=ORIENTED_EDGE('',*,*,#11929,.T.);
#16566=ORIENTED_EDGE('',*,*,#11794,.T.);
#16567=ORIENTED_EDGE('',*,*,#11930,.T.);
#16568=ORIENTED_EDGE('',*,*,#11790,.T.);
#16569=ORIENTED_EDGE('',*,*,#11931,.T.);
#16570=ORIENTED_EDGE('',*,*,#11786,.T.);
#16571=ORIENTED_EDGE('',*,*,#11932,.T.);
#16572=ORIENTED_EDGE('',*,*,#11782,.T.);
#16573=ORIENTED_EDGE('',*,*,#11933,.T.);
#16574=ORIENTED_EDGE('',*,*,#11778,.T.);
#16575=ORIENTED_EDGE('',*,*,#11934,.T.);
#16576=ORIENTED_EDGE('',*,*,#11774,.T.);
#16577=ORIENTED_EDGE('',*,*,#11935,.T.);
#16578=ORIENTED_EDGE('',*,*,#11770,.T.);
#16579=ORIENTED_EDGE('',*,*,#11936,.T.);
#16580=ORIENTED_EDGE('',*,*,#11766,.T.);
#16581=ORIENTED_EDGE('',*,*,#11937,.T.);
#16582=ORIENTED_EDGE('',*,*,#11762,.T.);
#16583=ORIENTED_EDGE('',*,*,#11938,.T.);
#16584=ORIENTED_EDGE('',*,*,#11758,.T.);
#16585=ORIENTED_EDGE('',*,*,#11939,.T.);
#16586=ORIENTED_EDGE('',*,*,#11754,.T.);
#16587=ORIENTED_EDGE('',*,*,#11940,.T.);
#16588=ORIENTED_EDGE('',*,*,#11750,.T.);
#16589=ORIENTED_EDGE('',*,*,#11941,.T.);
#16590=ORIENTED_EDGE('',*,*,#11746,.T.);
#16591=ORIENTED_EDGE('',*,*,#11942,.T.);
#16592=ORIENTED_EDGE('',*,*,#11742,.T.);
#16593=ORIENTED_EDGE('',*,*,#11943,.T.);
#16594=ORIENTED_EDGE('',*,*,#11738,.T.);
#16595=ORIENTED_EDGE('',*,*,#11944,.T.);
#16596=ORIENTED_EDGE('',*,*,#11734,.T.);
#16597=ORIENTED_EDGE('',*,*,#11945,.T.);
#16598=ORIENTED_EDGE('',*,*,#11730,.T.);
#16599=ORIENTED_EDGE('',*,*,#11946,.T.);
#16600=ORIENTED_EDGE('',*,*,#11947,.T.);
#16601=ORIENTED_EDGE('',*,*,#11725,.T.);
#16602=ORIENTED_EDGE('',*,*,#11948,.T.);
#16603=ORIENTED_EDGE('',*,*,#11949,.T.);
#16604=ORIENTED_EDGE('',*,*,#11901,.F.);
#16605=ORIENTED_EDGE('',*,*,#11899,.T.);
#16606=ORIENTED_EDGE('',*,*,#11903,.F.);
#16607=ORIENTED_EDGE('',*,*,#11950,.T.);
#16608=ORIENTED_EDGE('',*,*,#11951,.T.);
#16609=ORIENTED_EDGE('',*,*,#11895,.T.);
#16610=ORIENTED_EDGE('',*,*,#11904,.F.);
#16611=ORIENTED_EDGE('',*,*,#11897,.T.);
#16612=ORIENTED_EDGE('',*,*,#11952,.T.);
#16613=ORIENTED_EDGE('',*,*,#11891,.T.);
#16614=ORIENTED_EDGE('',*,*,#11905,.F.);
#16615=ORIENTED_EDGE('',*,*,#11893,.T.);
#16616=ORIENTED_EDGE('',*,*,#11953,.T.);
#16617=ORIENTED_EDGE('',*,*,#11887,.T.);
#16618=ORIENTED_EDGE('',*,*,#11906,.F.);
#16619=ORIENTED_EDGE('',*,*,#11889,.T.);
#16620=ORIENTED_EDGE('',*,*,#11954,.T.);
#16621=ORIENTED_EDGE('',*,*,#11883,.T.);
#16622=ORIENTED_EDGE('',*,*,#11907,.F.);
#16623=ORIENTED_EDGE('',*,*,#11885,.T.);
#16624=ORIENTED_EDGE('',*,*,#11955,.T.);
#16625=ORIENTED_EDGE('',*,*,#11879,.T.);
#16626=ORIENTED_EDGE('',*,*,#11908,.F.);
#16627=ORIENTED_EDGE('',*,*,#11881,.T.);
#16628=ORIENTED_EDGE('',*,*,#11956,.T.);
#16629=ORIENTED_EDGE('',*,*,#11875,.T.);
#16630=ORIENTED_EDGE('',*,*,#11909,.F.);
#16631=ORIENTED_EDGE('',*,*,#11877,.T.);
#16632=ORIENTED_EDGE('',*,*,#11957,.T.);
#16633=ORIENTED_EDGE('',*,*,#11871,.T.);
#16634=ORIENTED_EDGE('',*,*,#11910,.F.);
#16635=ORIENTED_EDGE('',*,*,#11873,.T.);
#16636=ORIENTED_EDGE('',*,*,#11958,.T.);
#16637=ORIENTED_EDGE('',*,*,#11867,.T.);
#16638=ORIENTED_EDGE('',*,*,#11911,.F.);
#16639=ORIENTED_EDGE('',*,*,#11869,.T.);
#16640=ORIENTED_EDGE('',*,*,#11959,.T.);
#16641=ORIENTED_EDGE('',*,*,#11863,.T.);
#16642=ORIENTED_EDGE('',*,*,#11912,.F.);
#16643=ORIENTED_EDGE('',*,*,#11865,.T.);
#16644=ORIENTED_EDGE('',*,*,#11960,.T.);
#16645=ORIENTED_EDGE('',*,*,#11859,.T.);
#16646=ORIENTED_EDGE('',*,*,#11913,.F.);
#16647=ORIENTED_EDGE('',*,*,#11861,.T.);
#16648=ORIENTED_EDGE('',*,*,#11961,.T.);
#16649=ORIENTED_EDGE('',*,*,#11855,.T.);
#16650=ORIENTED_EDGE('',*,*,#11914,.F.);
#16651=ORIENTED_EDGE('',*,*,#11857,.T.);
#16652=ORIENTED_EDGE('',*,*,#11962,.T.);
#16653=ORIENTED_EDGE('',*,*,#11851,.T.);
#16654=ORIENTED_EDGE('',*,*,#11915,.F.);
#16655=ORIENTED_EDGE('',*,*,#11853,.T.);
#16656=ORIENTED_EDGE('',*,*,#11963,.T.);
#16657=ORIENTED_EDGE('',*,*,#11847,.T.);
#16658=ORIENTED_EDGE('',*,*,#11916,.F.);
#16659=ORIENTED_EDGE('',*,*,#11849,.T.);
#16660=ORIENTED_EDGE('',*,*,#11964,.T.);
#16661=ORIENTED_EDGE('',*,*,#11843,.T.);
#16662=ORIENTED_EDGE('',*,*,#11917,.F.);
#16663=ORIENTED_EDGE('',*,*,#11845,.T.);
#16664=ORIENTED_EDGE('',*,*,#11965,.T.);
#16665=ORIENTED_EDGE('',*,*,#11839,.T.);
#16666=ORIENTED_EDGE('',*,*,#11918,.F.);
#16667=ORIENTED_EDGE('',*,*,#11841,.T.);
#16668=ORIENTED_EDGE('',*,*,#11966,.T.);
#16669=ORIENTED_EDGE('',*,*,#11835,.T.);
#16670=ORIENTED_EDGE('',*,*,#11919,.F.);
#16671=ORIENTED_EDGE('',*,*,#11837,.T.);
#16672=ORIENTED_EDGE('',*,*,#11967,.T.);
#16673=ORIENTED_EDGE('',*,*,#11831,.T.);
#16674=ORIENTED_EDGE('',*,*,#11920,.F.);
#16675=ORIENTED_EDGE('',*,*,#11833,.T.);
#16676=ORIENTED_EDGE('',*,*,#11968,.T.);
#16677=ORIENTED_EDGE('',*,*,#11827,.T.);
#16678=ORIENTED_EDGE('',*,*,#11921,.F.);
#16679=ORIENTED_EDGE('',*,*,#11829,.T.);
#16680=ORIENTED_EDGE('',*,*,#11969,.T.);
#16681=ORIENTED_EDGE('',*,*,#11823,.T.);
#16682=ORIENTED_EDGE('',*,*,#11922,.F.);
#16683=ORIENTED_EDGE('',*,*,#11825,.T.);
#16684=ORIENTED_EDGE('',*,*,#11970,.T.);
#16685=ORIENTED_EDGE('',*,*,#11819,.T.);
#16686=ORIENTED_EDGE('',*,*,#11923,.F.);
#16687=ORIENTED_EDGE('',*,*,#11821,.T.);
#16688=ORIENTED_EDGE('',*,*,#11971,.T.);
#16689=ORIENTED_EDGE('',*,*,#11815,.T.);
#16690=ORIENTED_EDGE('',*,*,#11924,.F.);
#16691=ORIENTED_EDGE('',*,*,#11817,.T.);
#16692=ORIENTED_EDGE('',*,*,#11972,.T.);
#16693=ORIENTED_EDGE('',*,*,#11811,.T.);
#16694=ORIENTED_EDGE('',*,*,#11925,.F.);
#16695=ORIENTED_EDGE('',*,*,#11813,.T.);
#16696=ORIENTED_EDGE('',*,*,#11973,.T.);
#16697=ORIENTED_EDGE('',*,*,#11807,.T.);
#16698=ORIENTED_EDGE('',*,*,#11926,.F.);
#16699=ORIENTED_EDGE('',*,*,#11809,.T.);
#16700=ORIENTED_EDGE('',*,*,#11974,.T.);
#16701=ORIENTED_EDGE('',*,*,#11803,.T.);
#16702=ORIENTED_EDGE('',*,*,#11927,.F.);
#16703=ORIENTED_EDGE('',*,*,#11805,.T.);
#16704=ORIENTED_EDGE('',*,*,#11975,.T.);
#16705=ORIENTED_EDGE('',*,*,#11799,.T.);
#16706=ORIENTED_EDGE('',*,*,#11928,.F.);
#16707=ORIENTED_EDGE('',*,*,#11801,.T.);
#16708=ORIENTED_EDGE('',*,*,#11976,.T.);
#16709=ORIENTED_EDGE('',*,*,#11795,.T.);
#16710=ORIENTED_EDGE('',*,*,#11929,.F.);
#16711=ORIENTED_EDGE('',*,*,#11797,.T.);
#16712=ORIENTED_EDGE('',*,*,#11977,.T.);
#16713=ORIENTED_EDGE('',*,*,#11791,.T.);
#16714=ORIENTED_EDGE('',*,*,#11930,.F.);
#16715=ORIENTED_EDGE('',*,*,#11793,.T.);
#16716=ORIENTED_EDGE('',*,*,#11978,.T.);
#16717=ORIENTED_EDGE('',*,*,#11787,.T.);
#16718=ORIENTED_EDGE('',*,*,#11931,.F.);
#16719=ORIENTED_EDGE('',*,*,#11789,.T.);
#16720=ORIENTED_EDGE('',*,*,#11979,.T.);
#16721=ORIENTED_EDGE('',*,*,#11783,.T.);
#16722=ORIENTED_EDGE('',*,*,#11932,.F.);
#16723=ORIENTED_EDGE('',*,*,#11785,.T.);
#16724=ORIENTED_EDGE('',*,*,#11980,.T.);
#16725=ORIENTED_EDGE('',*,*,#11779,.T.);
#16726=ORIENTED_EDGE('',*,*,#11933,.F.);
#16727=ORIENTED_EDGE('',*,*,#11781,.T.);
#16728=ORIENTED_EDGE('',*,*,#11981,.T.);
#16729=ORIENTED_EDGE('',*,*,#11775,.T.);
#16730=ORIENTED_EDGE('',*,*,#11934,.F.);
#16731=ORIENTED_EDGE('',*,*,#11777,.T.);
#16732=ORIENTED_EDGE('',*,*,#11982,.T.);
#16733=ORIENTED_EDGE('',*,*,#11771,.T.);
#16734=ORIENTED_EDGE('',*,*,#11935,.F.);
#16735=ORIENTED_EDGE('',*,*,#11773,.T.);
#16736=ORIENTED_EDGE('',*,*,#11983,.T.);
#16737=ORIENTED_EDGE('',*,*,#11767,.T.);
#16738=ORIENTED_EDGE('',*,*,#11936,.F.);
#16739=ORIENTED_EDGE('',*,*,#11769,.T.);
#16740=ORIENTED_EDGE('',*,*,#11984,.T.);
#16741=ORIENTED_EDGE('',*,*,#11763,.T.);
#16742=ORIENTED_EDGE('',*,*,#11937,.F.);
#16743=ORIENTED_EDGE('',*,*,#11765,.T.);
#16744=ORIENTED_EDGE('',*,*,#11985,.T.);
#16745=ORIENTED_EDGE('',*,*,#11759,.T.);
#16746=ORIENTED_EDGE('',*,*,#11938,.F.);
#16747=ORIENTED_EDGE('',*,*,#11761,.T.);
#16748=ORIENTED_EDGE('',*,*,#11986,.T.);
#16749=ORIENTED_EDGE('',*,*,#11755,.T.);
#16750=ORIENTED_EDGE('',*,*,#11939,.F.);
#16751=ORIENTED_EDGE('',*,*,#11757,.T.);
#16752=ORIENTED_EDGE('',*,*,#11987,.T.);
#16753=ORIENTED_EDGE('',*,*,#11751,.T.);
#16754=ORIENTED_EDGE('',*,*,#11940,.F.);
#16755=ORIENTED_EDGE('',*,*,#11753,.T.);
#16756=ORIENTED_EDGE('',*,*,#11988,.T.);
#16757=ORIENTED_EDGE('',*,*,#11747,.T.);
#16758=ORIENTED_EDGE('',*,*,#11941,.F.);
#16759=ORIENTED_EDGE('',*,*,#11749,.T.);
#16760=ORIENTED_EDGE('',*,*,#11989,.T.);
#16761=ORIENTED_EDGE('',*,*,#11743,.T.);
#16762=ORIENTED_EDGE('',*,*,#11942,.F.);
#16763=ORIENTED_EDGE('',*,*,#11745,.T.);
#16764=ORIENTED_EDGE('',*,*,#11990,.T.);
#16765=ORIENTED_EDGE('',*,*,#11739,.T.);
#16766=ORIENTED_EDGE('',*,*,#11943,.F.);
#16767=ORIENTED_EDGE('',*,*,#11741,.T.);
#16768=ORIENTED_EDGE('',*,*,#11991,.T.);
#16769=ORIENTED_EDGE('',*,*,#11735,.T.);
#16770=ORIENTED_EDGE('',*,*,#11944,.F.);
#16771=ORIENTED_EDGE('',*,*,#11737,.T.);
#16772=ORIENTED_EDGE('',*,*,#11992,.T.);
#16773=ORIENTED_EDGE('',*,*,#11731,.T.);
#16774=ORIENTED_EDGE('',*,*,#11945,.F.);
#16775=ORIENTED_EDGE('',*,*,#11733,.T.);
#16776=ORIENTED_EDGE('',*,*,#11993,.T.);
#16777=ORIENTED_EDGE('',*,*,#11950,.F.);
#16778=ORIENTED_EDGE('',*,*,#11902,.F.);
#16779=ORIENTED_EDGE('',*,*,#11949,.F.);
#16780=ORIENTED_EDGE('',*,*,#11994,.F.);
#16781=ORIENTED_EDGE('',*,*,#11728,.T.);
#16782=ORIENTED_EDGE('',*,*,#11995,.F.);
#16783=ORIENTED_EDGE('',*,*,#11732,.T.);
#16784=ORIENTED_EDGE('',*,*,#11993,.F.);
#16785=ORIENTED_EDGE('',*,*,#11736,.T.);
#16786=ORIENTED_EDGE('',*,*,#11992,.F.);
#16787=ORIENTED_EDGE('',*,*,#11740,.T.);
#16788=ORIENTED_EDGE('',*,*,#11991,.F.);
#16789=ORIENTED_EDGE('',*,*,#11744,.T.);
#16790=ORIENTED_EDGE('',*,*,#11990,.F.);
#16791=ORIENTED_EDGE('',*,*,#11748,.T.);
#16792=ORIENTED_EDGE('',*,*,#11989,.F.);
#16793=ORIENTED_EDGE('',*,*,#11752,.T.);
#16794=ORIENTED_EDGE('',*,*,#11988,.F.);
#16795=ORIENTED_EDGE('',*,*,#11756,.T.);
#16796=ORIENTED_EDGE('',*,*,#11987,.F.);
#16797=ORIENTED_EDGE('',*,*,#11760,.T.);
#16798=ORIENTED_EDGE('',*,*,#11986,.F.);
#16799=ORIENTED_EDGE('',*,*,#11764,.T.);
#16800=ORIENTED_EDGE('',*,*,#11985,.F.);
#16801=ORIENTED_EDGE('',*,*,#11768,.T.);
#16802=ORIENTED_EDGE('',*,*,#11984,.F.);
#16803=ORIENTED_EDGE('',*,*,#11772,.T.);
#16804=ORIENTED_EDGE('',*,*,#11983,.F.);
#16805=ORIENTED_EDGE('',*,*,#11776,.T.);
#16806=ORIENTED_EDGE('',*,*,#11982,.F.);
#16807=ORIENTED_EDGE('',*,*,#11780,.T.);
#16808=ORIENTED_EDGE('',*,*,#11981,.F.);
#16809=ORIENTED_EDGE('',*,*,#11784,.T.);
#16810=ORIENTED_EDGE('',*,*,#11980,.F.);
#16811=ORIENTED_EDGE('',*,*,#11788,.T.);
#16812=ORIENTED_EDGE('',*,*,#11979,.F.);
#16813=ORIENTED_EDGE('',*,*,#11792,.T.);
#16814=ORIENTED_EDGE('',*,*,#11978,.F.);
#16815=ORIENTED_EDGE('',*,*,#11796,.T.);
#16816=ORIENTED_EDGE('',*,*,#11977,.F.);
#16817=ORIENTED_EDGE('',*,*,#11800,.T.);
#16818=ORIENTED_EDGE('',*,*,#11976,.F.);
#16819=ORIENTED_EDGE('',*,*,#11804,.T.);
#16820=ORIENTED_EDGE('',*,*,#11975,.F.);
#16821=ORIENTED_EDGE('',*,*,#11808,.T.);
#16822=ORIENTED_EDGE('',*,*,#11974,.F.);
#16823=ORIENTED_EDGE('',*,*,#11812,.T.);
#16824=ORIENTED_EDGE('',*,*,#11973,.F.);
#16825=ORIENTED_EDGE('',*,*,#11816,.T.);
#16826=ORIENTED_EDGE('',*,*,#11972,.F.);
#16827=ORIENTED_EDGE('',*,*,#11820,.T.);
#16828=ORIENTED_EDGE('',*,*,#11971,.F.);
#16829=ORIENTED_EDGE('',*,*,#11824,.T.);
#16830=ORIENTED_EDGE('',*,*,#11970,.F.);
#16831=ORIENTED_EDGE('',*,*,#11828,.T.);
#16832=ORIENTED_EDGE('',*,*,#11969,.F.);
#16833=ORIENTED_EDGE('',*,*,#11832,.T.);
#16834=ORIENTED_EDGE('',*,*,#11968,.F.);
#16835=ORIENTED_EDGE('',*,*,#11836,.T.);
#16836=ORIENTED_EDGE('',*,*,#11967,.F.);
#16837=ORIENTED_EDGE('',*,*,#11840,.T.);
#16838=ORIENTED_EDGE('',*,*,#11966,.F.);
#16839=ORIENTED_EDGE('',*,*,#11844,.T.);
#16840=ORIENTED_EDGE('',*,*,#11965,.F.);
#16841=ORIENTED_EDGE('',*,*,#11848,.T.);
#16842=ORIENTED_EDGE('',*,*,#11964,.F.);
#16843=ORIENTED_EDGE('',*,*,#11852,.T.);
#16844=ORIENTED_EDGE('',*,*,#11963,.F.);
#16845=ORIENTED_EDGE('',*,*,#11856,.T.);
#16846=ORIENTED_EDGE('',*,*,#11962,.F.);
#16847=ORIENTED_EDGE('',*,*,#11860,.T.);
#16848=ORIENTED_EDGE('',*,*,#11961,.F.);
#16849=ORIENTED_EDGE('',*,*,#11864,.T.);
#16850=ORIENTED_EDGE('',*,*,#11960,.F.);
#16851=ORIENTED_EDGE('',*,*,#11868,.T.);
#16852=ORIENTED_EDGE('',*,*,#11959,.F.);
#16853=ORIENTED_EDGE('',*,*,#11872,.T.);
#16854=ORIENTED_EDGE('',*,*,#11958,.F.);
#16855=ORIENTED_EDGE('',*,*,#11876,.T.);
#16856=ORIENTED_EDGE('',*,*,#11957,.F.);
#16857=ORIENTED_EDGE('',*,*,#11880,.T.);
#16858=ORIENTED_EDGE('',*,*,#11956,.F.);
#16859=ORIENTED_EDGE('',*,*,#11884,.T.);
#16860=ORIENTED_EDGE('',*,*,#11955,.F.);
#16861=ORIENTED_EDGE('',*,*,#11888,.T.);
#16862=ORIENTED_EDGE('',*,*,#11954,.F.);
#16863=ORIENTED_EDGE('',*,*,#11892,.T.);
#16864=ORIENTED_EDGE('',*,*,#11953,.F.);
#16865=ORIENTED_EDGE('',*,*,#11896,.T.);
#16866=ORIENTED_EDGE('',*,*,#11952,.F.);
#16867=ORIENTED_EDGE('',*,*,#11900,.T.);
#16868=ORIENTED_EDGE('',*,*,#11951,.F.);
#16869=ORIENTED_EDGE('',*,*,#11994,.T.);
#16870=ORIENTED_EDGE('',*,*,#11948,.F.);
#16871=ORIENTED_EDGE('',*,*,#11996,.F.);
#16872=ORIENTED_EDGE('',*,*,#11727,.T.);
#16873=ORIENTED_EDGE('',*,*,#11946,.F.);
#16874=ORIENTED_EDGE('',*,*,#11729,.T.);
#16875=ORIENTED_EDGE('',*,*,#11995,.T.);
#16876=ORIENTED_EDGE('',*,*,#11996,.T.);
#16877=ORIENTED_EDGE('',*,*,#11997,.T.);
#16878=ORIENTED_EDGE('',*,*,#11947,.F.);
#16879=ORIENTED_EDGE('',*,*,#11997,.F.);
#19169=ADVANCED_FACE('',(#5453),#4588,.F.);
#19170=ADVANCED_FACE('',(#5454),#4589,.F.);
#19171=ADVANCED_FACE('',(#5455),#4590,.F.);
#19172=ADVANCED_FACE('',(#5456),#4591,.F.);
#19173=ADVANCED_FACE('',(#5457),#4592,.F.);
#19174=ADVANCED_FACE('',(#5458),#4593,.F.);
#19175=ADVANCED_FACE('',(#5459),#4594,.F.);
#19176=ADVANCED_FACE('',(#5460),#4595,.F.);
#19177=ADVANCED_FACE('',(#5461),#4596,.F.);
#19178=ADVANCED_FACE('',(#5462),#4597,.F.);
#19179=ADVANCED_FACE('',(#5463),#4598,.F.);
#19180=ADVANCED_FACE('',(#5464),#4599,.F.);
#19181=ADVANCED_FACE('',(#5465),#4600,.F.);
#19182=ADVANCED_FACE('',(#5466),#4601,.F.);
#19183=ADVANCED_FACE('',(#5467),#4602,.F.);
#19184=ADVANCED_FACE('',(#5468),#4603,.F.);
#19185=ADVANCED_FACE('',(#5469),#4604,.F.);
#19186=ADVANCED_FACE('',(#5470),#4605,.F.);
#19187=ADVANCED_FACE('',(#5471),#4606,.F.);
#19188=ADVANCED_FACE('',(#5472),#4607,.F.);
#19189=ADVANCED_FACE('',(#5473),#4608,.F.);
#19190=ADVANCED_FACE('',(#5474),#4609,.F.);
#19191=ADVANCED_FACE('',(#5475),#4610,.F.);
#19192=ADVANCED_FACE('',(#5476),#4611,.F.);
#19193=ADVANCED_FACE('',(#5477),#4612,.F.);
#19194=ADVANCED_FACE('',(#5478),#4613,.F.);
#19195=ADVANCED_FACE('',(#5479),#4614,.F.);
#19196=ADVANCED_FACE('',(#5480),#4615,.F.);
#19197=ADVANCED_FACE('',(#5481),#4616,.F.);
#19198=ADVANCED_FACE('',(#5482),#4617,.F.);
#19199=ADVANCED_FACE('',(#5483),#4618,.F.);
#19200=ADVANCED_FACE('',(#5484),#4619,.F.);
#19201=ADVANCED_FACE('',(#5485),#4620,.F.);
#19202=ADVANCED_FACE('',(#5486),#4621,.F.);
#19203=ADVANCED_FACE('',(#5487),#4622,.F.);
#19204=ADVANCED_FACE('',(#5488),#4623,.F.);
#19205=ADVANCED_FACE('',(#5489),#4624,.F.);
#19206=ADVANCED_FACE('',(#5490),#4625,.F.);
#19207=ADVANCED_FACE('',(#5491),#4626,.F.);
#19208=ADVANCED_FACE('',(#5492),#4627,.F.);
#19209=ADVANCED_FACE('',(#5493),#4628,.F.);
#19210=ADVANCED_FACE('',(#5494),#4629,.F.);
#19211=ADVANCED_FACE('',(#5495),#4630,.F.);
#19212=ADVANCED_FACE('',(#5496),#4631,.F.);
#19213=ADVANCED_FACE('',(#5497,#558),#925,.T.);
#19214=ADVANCED_FACE('',(#5498),#4632,.T.);
#19215=ADVANCED_FACE('',(#5499),#4633,.T.);
#19216=ADVANCED_FACE('',(#5500),#4634,.T.);
#19217=ADVANCED_FACE('',(#5501),#4635,.T.);
#19218=ADVANCED_FACE('',(#5502),#4636,.T.);
#19219=ADVANCED_FACE('',(#5503),#4637,.T.);
#19220=ADVANCED_FACE('',(#5504),#4638,.T.);
#19221=ADVANCED_FACE('',(#5505),#4639,.T.);
#19222=ADVANCED_FACE('',(#5506),#4640,.T.);
#19223=ADVANCED_FACE('',(#5507),#4641,.T.);
#19224=ADVANCED_FACE('',(#5508),#4642,.T.);
#19225=ADVANCED_FACE('',(#5509),#4643,.T.);
#19226=ADVANCED_FACE('',(#5510),#4644,.T.);
#19227=ADVANCED_FACE('',(#5511),#4645,.T.);
#19228=ADVANCED_FACE('',(#5512),#4646,.T.);
#19229=ADVANCED_FACE('',(#5513),#4647,.T.);
#19230=ADVANCED_FACE('',(#5514),#4648,.T.);
#19231=ADVANCED_FACE('',(#5515),#4649,.T.);
#19232=ADVANCED_FACE('',(#5516),#4650,.T.);
#19233=ADVANCED_FACE('',(#5517),#4651,.T.);
#19234=ADVANCED_FACE('',(#5518),#4652,.T.);
#19235=ADVANCED_FACE('',(#5519),#4653,.T.);
#19236=ADVANCED_FACE('',(#5520),#4654,.T.);
#19237=ADVANCED_FACE('',(#5521),#4655,.T.);
#19238=ADVANCED_FACE('',(#5522),#4656,.T.);
#19239=ADVANCED_FACE('',(#5523),#4657,.T.);
#19240=ADVANCED_FACE('',(#5524),#4658,.T.);
#19241=ADVANCED_FACE('',(#5525),#4659,.T.);
#19242=ADVANCED_FACE('',(#5526),#4660,.T.);
#19243=ADVANCED_FACE('',(#5527),#4661,.T.);
#19244=ADVANCED_FACE('',(#5528),#4662,.T.);
#19245=ADVANCED_FACE('',(#5529),#4663,.T.);
#19246=ADVANCED_FACE('',(#5530),#4664,.T.);
#19247=ADVANCED_FACE('',(#5531),#4665,.T.);
#19248=ADVANCED_FACE('',(#5532),#4666,.T.);
#19249=ADVANCED_FACE('',(#5533),#4667,.T.);
#19250=ADVANCED_FACE('',(#5534),#4668,.T.);
#19251=ADVANCED_FACE('',(#5535),#4669,.T.);
#19252=ADVANCED_FACE('',(#5536),#4670,.T.);
#19253=ADVANCED_FACE('',(#5537),#4671,.T.);
#19254=ADVANCED_FACE('',(#5538),#4672,.T.);
#19255=ADVANCED_FACE('',(#5539),#4673,.T.);
#19256=ADVANCED_FACE('',(#5540),#4674,.T.);
#19257=ADVANCED_FACE('',(#5541),#4675,.T.);
#19258=ADVANCED_FACE('',(#5542),#4676,.F.);
#19259=ADVANCED_FACE('',(#5543,#559),#926,.F.);
#19260=ADVANCED_FACE('',(#5544),#4677,.T.);
#19261=ADVANCED_FACE('',(#5545),#4678,.F.);
#19574=CLOSED_SHELL('',(#19169,#19170,#19171,#19172,#19173,#19174,#19175,
#19176,#19177,#19178,#19179,#19180,#19181,#19182,#19183,#19184,#19185,#19186,
#19187,#19188,#19189,#19190,#19191,#19192,#19193,#19194,#19195,#19196,#19197,
#19198,#19199,#19200,#19201,#19202,#19203,#19204,#19205,#19206,#19207,#19208,
#19209,#19210,#19211,#19212,#19213,#19214,#19215,#19216,#19217,#19218,#19219,
#19220,#19221,#19222,#19223,#19224,#19225,#19226,#19227,#19228,#19229,#19230,
#19231,#19232,#19233,#19234,#19235,#19236,#19237,#19238,#19239,#19240,#19241,
#19242,#19243,#19244,#19245,#19246,#19247,#19248,#19249,#19250,#19251,#19252,
#19253,#19254,#19255,#19256,#19257,#19258,#19259,#19260,#19261));
#21374=AXIS2_PLACEMENT_3D('',#32380,#26104,#26105);
#21375=AXIS2_PLACEMENT_3D('',#32381,#26106,#26107);
#21376=AXIS2_PLACEMENT_3D('',#32386,#26109,#26110);
#21377=AXIS2_PLACEMENT_3D('',#32389,#26112,#26113);
#21378=AXIS2_PLACEMENT_3D('',#32390,#26114,#26115);
#21379=AXIS2_PLACEMENT_3D('',#32395,#26117,#26118);
#21380=AXIS2_PLACEMENT_3D('',#32398,#26120,#26121);
#21381=AXIS2_PLACEMENT_3D('',#32399,#26122,#26123);
#21382=AXIS2_PLACEMENT_3D('',#32404,#26125,#26126);
#21383=AXIS2_PLACEMENT_3D('',#32407,#26128,#26129);
#21384=AXIS2_PLACEMENT_3D('',#32408,#26130,#26131);
#21385=AXIS2_PLACEMENT_3D('',#32413,#26133,#26134);
#21386=AXIS2_PLACEMENT_3D('',#32416,#26136,#26137);
#21387=AXIS2_PLACEMENT_3D('',#32417,#26138,#26139);
#21388=AXIS2_PLACEMENT_3D('',#32422,#26141,#26142);
#21389=AXIS2_PLACEMENT_3D('',#32425,#26144,#26145);
#21390=AXIS2_PLACEMENT_3D('',#32426,#26146,#26147);
#21391=AXIS2_PLACEMENT_3D('',#32431,#26149,#26150);
#21392=AXIS2_PLACEMENT_3D('',#32434,#26152,#26153);
#21393=AXIS2_PLACEMENT_3D('',#32435,#26154,#26155);
#21394=AXIS2_PLACEMENT_3D('',#32440,#26157,#26158);
#21395=AXIS2_PLACEMENT_3D('',#32443,#26160,#26161);
#21396=AXIS2_PLACEMENT_3D('',#32444,#26162,#26163);
#21397=AXIS2_PLACEMENT_3D('',#32449,#26165,#26166);
#21398=AXIS2_PLACEMENT_3D('',#32452,#26168,#26169);
#21399=AXIS2_PLACEMENT_3D('',#32453,#26170,#26171);
#21400=AXIS2_PLACEMENT_3D('',#32458,#26173,#26174);
#21401=AXIS2_PLACEMENT_3D('',#32461,#26176,#26177);
#21402=AXIS2_PLACEMENT_3D('',#32462,#26178,#26179);
#21403=AXIS2_PLACEMENT_3D('',#32467,#26181,#26182);
#21404=AXIS2_PLACEMENT_3D('',#32470,#26184,#26185);
#21405=AXIS2_PLACEMENT_3D('',#32471,#26186,#26187);
#21406=AXIS2_PLACEMENT_3D('',#32476,#26189,#26190);
#21407=AXIS2_PLACEMENT_3D('',#32479,#26192,#26193);
#21408=AXIS2_PLACEMENT_3D('',#32480,#26194,#26195);
#21409=AXIS2_PLACEMENT_3D('',#32485,#26197,#26198);
#21410=AXIS2_PLACEMENT_3D('',#32488,#26200,#26201);
#21411=AXIS2_PLACEMENT_3D('',#32489,#26202,#26203);
#21412=AXIS2_PLACEMENT_3D('',#32494,#26205,#26206);
#21413=AXIS2_PLACEMENT_3D('',#32497,#26208,#26209);
#21414=AXIS2_PLACEMENT_3D('',#32498,#26210,#26211);
#21415=AXIS2_PLACEMENT_3D('',#32503,#26213,#26214);
#21416=AXIS2_PLACEMENT_3D('',#32506,#26216,#26217);
#21417=AXIS2_PLACEMENT_3D('',#32507,#26218,#26219);
#21418=AXIS2_PLACEMENT_3D('',#32512,#26221,#26222);
#21419=AXIS2_PLACEMENT_3D('',#32515,#26224,#26225);
#21420=AXIS2_PLACEMENT_3D('',#32516,#26226,#26227);
#21421=AXIS2_PLACEMENT_3D('',#32521,#26229,#26230);
#21422=AXIS2_PLACEMENT_3D('',#32524,#26232,#26233);
#21423=AXIS2_PLACEMENT_3D('',#32525,#26234,#26235);
#21424=AXIS2_PLACEMENT_3D('',#32530,#26237,#26238);
#21425=AXIS2_PLACEMENT_3D('',#32533,#26240,#26241);
#21426=AXIS2_PLACEMENT_3D('',#32534,#26242,#26243);
#21427=AXIS2_PLACEMENT_3D('',#32539,#26245,#26246);
#21428=AXIS2_PLACEMENT_3D('',#32542,#26248,#26249);
#21429=AXIS2_PLACEMENT_3D('',#32543,#26250,#26251);
#21430=AXIS2_PLACEMENT_3D('',#32548,#26253,#26254);
#21431=AXIS2_PLACEMENT_3D('',#32551,#26256,#26257);
#21432=AXIS2_PLACEMENT_3D('',#32552,#26258,#26259);
#21433=AXIS2_PLACEMENT_3D('',#32557,#26261,#26262);
#21434=AXIS2_PLACEMENT_3D('',#32560,#26264,#26265);
#21435=AXIS2_PLACEMENT_3D('',#32561,#26266,#26267);
#21436=AXIS2_PLACEMENT_3D('',#32566,#26269,#26270);
#21437=AXIS2_PLACEMENT_3D('',#32569,#26272,#26273);
#21438=AXIS2_PLACEMENT_3D('',#32570,#26274,#26275);
#21439=AXIS2_PLACEMENT_3D('',#32575,#26277,#26278);
#21440=AXIS2_PLACEMENT_3D('',#32578,#26280,#26281);
#21441=AXIS2_PLACEMENT_3D('',#32579,#26282,#26283);
#21442=AXIS2_PLACEMENT_3D('',#32584,#26285,#26286);
#21443=AXIS2_PLACEMENT_3D('',#32587,#26288,#26289);
#21444=AXIS2_PLACEMENT_3D('',#32588,#26290,#26291);
#21445=AXIS2_PLACEMENT_3D('',#32593,#26293,#26294);
#21446=AXIS2_PLACEMENT_3D('',#32596,#26296,#26297);
#21447=AXIS2_PLACEMENT_3D('',#32597,#26298,#26299);
#21448=AXIS2_PLACEMENT_3D('',#32602,#26301,#26302);
#21449=AXIS2_PLACEMENT_3D('',#32605,#26304,#26305);
#21450=AXIS2_PLACEMENT_3D('',#32606,#26306,#26307);
#21451=AXIS2_PLACEMENT_3D('',#32611,#26309,#26310);
#21452=AXIS2_PLACEMENT_3D('',#32614,#26312,#26313);
#21453=AXIS2_PLACEMENT_3D('',#32615,#26314,#26315);
#21454=AXIS2_PLACEMENT_3D('',#32620,#26317,#26318);
#21455=AXIS2_PLACEMENT_3D('',#32623,#26320,#26321);
#21456=AXIS2_PLACEMENT_3D('',#32624,#26322,#26323);
#21457=AXIS2_PLACEMENT_3D('',#32629,#26325,#26326);
#21458=AXIS2_PLACEMENT_3D('',#32632,#26328,#26329);
#21459=AXIS2_PLACEMENT_3D('',#32633,#26330,#26331);
#21460=AXIS2_PLACEMENT_3D('',#32638,#26333,#26334);
#21461=AXIS2_PLACEMENT_3D('',#32641,#26336,#26337);
#21462=AXIS2_PLACEMENT_3D('',#32642,#26338,#26339);
#21463=AXIS2_PLACEMENT_3D('',#32647,#26341,#26342);
#21464=AXIS2_PLACEMENT_3D('',#32650,#26344,#26345);
#21465=AXIS2_PLACEMENT_3D('',#32651,#26346,#26347);
#21466=AXIS2_PLACEMENT_3D('',#32656,#26349,#26350);
#21467=AXIS2_PLACEMENT_3D('',#32659,#26352,#26353);
#21468=AXIS2_PLACEMENT_3D('',#32660,#26354,#26355);
#21469=AXIS2_PLACEMENT_3D('',#32665,#26357,#26358);
#21470=AXIS2_PLACEMENT_3D('',#32668,#26360,#26361);
#21471=AXIS2_PLACEMENT_3D('',#32669,#26362,#26363);
#21472=AXIS2_PLACEMENT_3D('',#32674,#26365,#26366);
#21473=AXIS2_PLACEMENT_3D('',#32677,#26368,#26369);
#21474=AXIS2_PLACEMENT_3D('',#32678,#26370,#26371);
#21475=AXIS2_PLACEMENT_3D('',#32683,#26373,#26374);
#21476=AXIS2_PLACEMENT_3D('',#32686,#26376,#26377);
#21477=AXIS2_PLACEMENT_3D('',#32687,#26378,#26379);
#21478=AXIS2_PLACEMENT_3D('',#32692,#26381,#26382);
#21479=AXIS2_PLACEMENT_3D('',#32695,#26384,#26385);
#21480=AXIS2_PLACEMENT_3D('',#32696,#26386,#26387);
#21481=AXIS2_PLACEMENT_3D('',#32701,#26389,#26390);
#21482=AXIS2_PLACEMENT_3D('',#32704,#26392,#26393);
#21483=AXIS2_PLACEMENT_3D('',#32705,#26394,#26395);
#21484=AXIS2_PLACEMENT_3D('',#32710,#26397,#26398);
#21485=AXIS2_PLACEMENT_3D('',#32713,#26400,#26401);
#21486=AXIS2_PLACEMENT_3D('',#32714,#26402,#26403);
#21487=AXIS2_PLACEMENT_3D('',#32719,#26405,#26406);
#21488=AXIS2_PLACEMENT_3D('',#32722,#26408,#26409);
#21489=AXIS2_PLACEMENT_3D('',#32723,#26410,#26411);
#21490=AXIS2_PLACEMENT_3D('',#32728,#26413,#26414);
#21491=AXIS2_PLACEMENT_3D('',#32731,#26416,#26417);
#21492=AXIS2_PLACEMENT_3D('',#32732,#26418,#26419);
#21493=AXIS2_PLACEMENT_3D('',#32737,#26421,#26422);
#21494=AXIS2_PLACEMENT_3D('',#32740,#26424,#26425);
#21495=AXIS2_PLACEMENT_3D('',#32741,#26426,#26427);
#21496=AXIS2_PLACEMENT_3D('',#32746,#26429,#26430);
#21497=AXIS2_PLACEMENT_3D('',#32749,#26432,#26433);
#21498=AXIS2_PLACEMENT_3D('',#32750,#26434,#26435);
#21499=AXIS2_PLACEMENT_3D('',#32755,#26437,#26438);
#21500=AXIS2_PLACEMENT_3D('',#32758,#26440,#26441);
#21501=AXIS2_PLACEMENT_3D('',#32759,#26442,#26443);
#21502=AXIS2_PLACEMENT_3D('',#32764,#26445,#26446);
#21503=AXIS2_PLACEMENT_3D('',#32767,#26448,#26449);
#21504=AXIS2_PLACEMENT_3D('',#32768,#26450,#26451);
#21505=AXIS2_PLACEMENT_3D('',#32773,#26453,#26454);
#21506=AXIS2_PLACEMENT_3D('',#32776,#26456,#26457);
#21507=AXIS2_PLACEMENT_3D('',#32777,#26458,#26459);
#21508=AXIS2_PLACEMENT_3D('',#32779,#26460,#26461);
#21509=AXIS2_PLACEMENT_3D('',#32781,#26462,#26463);
#21510=AXIS2_PLACEMENT_3D('',#32782,#26464,#26465);
#21511=AXIS2_PLACEMENT_3D('',#32783,#26466,#26467);
#21512=AXIS2_PLACEMENT_3D('',#32784,#26468,#26469);
#21513=AXIS2_PLACEMENT_3D('',#32785,#26470,#26471);
#21514=AXIS2_PLACEMENT_3D('',#32786,#26472,#26473);
#21515=AXIS2_PLACEMENT_3D('',#32787,#26474,#26475);
#21516=AXIS2_PLACEMENT_3D('',#32788,#26476,#26477);
#21517=AXIS2_PLACEMENT_3D('',#32789,#26478,#26479);
#21518=AXIS2_PLACEMENT_3D('',#32790,#26480,#26481);
#21519=AXIS2_PLACEMENT_3D('',#32791,#26482,#26483);
#21520=AXIS2_PLACEMENT_3D('',#32792,#26484,#26485);
#21521=AXIS2_PLACEMENT_3D('',#32793,#26486,#26487);
#21522=AXIS2_PLACEMENT_3D('',#32794,#26488,#26489);
#21523=AXIS2_PLACEMENT_3D('',#32795,#26490,#26491);
#21524=AXIS2_PLACEMENT_3D('',#32796,#26492,#26493);
#21525=AXIS2_PLACEMENT_3D('',#32797,#26494,#26495);
#21526=AXIS2_PLACEMENT_3D('',#32798,#26496,#26497);
#21527=AXIS2_PLACEMENT_3D('',#32799,#26498,#26499);
#21528=AXIS2_PLACEMENT_3D('',#32800,#26500,#26501);
#21529=AXIS2_PLACEMENT_3D('',#32801,#26502,#26503);
#21530=AXIS2_PLACEMENT_3D('',#32802,#26504,#26505);
#21531=AXIS2_PLACEMENT_3D('',#32803,#26506,#26507);
#21532=AXIS2_PLACEMENT_3D('',#32804,#26508,#26509);
#21533=AXIS2_PLACEMENT_3D('',#32805,#26510,#26511);
#21534=AXIS2_PLACEMENT_3D('',#32806,#26512,#26513);
#21535=AXIS2_PLACEMENT_3D('',#32807,#26514,#26515);
#21536=AXIS2_PLACEMENT_3D('',#32808,#26516,#26517);
#21537=AXIS2_PLACEMENT_3D('',#32809,#26518,#26519);
#21538=AXIS2_PLACEMENT_3D('',#32810,#26520,#26521);
#21539=AXIS2_PLACEMENT_3D('',#32811,#26522,#26523);
#21540=AXIS2_PLACEMENT_3D('',#32812,#26524,#26525);
#21541=AXIS2_PLACEMENT_3D('',#32813,#26526,#26527);
#21542=AXIS2_PLACEMENT_3D('',#32814,#26528,#26529);
#21543=AXIS2_PLACEMENT_3D('',#32815,#26530,#26531);
#21544=AXIS2_PLACEMENT_3D('',#32816,#26532,#26533);
#21545=AXIS2_PLACEMENT_3D('',#32817,#26534,#26535);
#21546=AXIS2_PLACEMENT_3D('',#32818,#26536,#26537);
#21547=AXIS2_PLACEMENT_3D('',#32819,#26538,#26539);
#21548=AXIS2_PLACEMENT_3D('',#32820,#26540,#26541);
#21549=AXIS2_PLACEMENT_3D('',#32821,#26542,#26543);
#21550=AXIS2_PLACEMENT_3D('',#32822,#26544,#26545);
#21551=AXIS2_PLACEMENT_3D('',#32823,#26546,#26547);
#21552=AXIS2_PLACEMENT_3D('',#32824,#26548,#26549);
#21553=AXIS2_PLACEMENT_3D('',#32825,#26550,#26551);
#21554=AXIS2_PLACEMENT_3D('',#32827,#26552,#26553);
#21555=AXIS2_PLACEMENT_3D('',#32828,#26554,#26555);
#21556=AXIS2_PLACEMENT_3D('',#32830,#26556,#26557);
#21557=AXIS2_PLACEMENT_3D('',#32832,#26559,#26560);
#21558=AXIS2_PLACEMENT_3D('',#32835,#26562,#26563);
#21559=AXIS2_PLACEMENT_3D('',#32836,#26564,#26565);
#21560=AXIS2_PLACEMENT_3D('',#32837,#26566,#26567);
#21561=AXIS2_PLACEMENT_3D('',#32838,#26568,#26569);
#21562=AXIS2_PLACEMENT_3D('',#32839,#26570,#26571);
#21563=AXIS2_PLACEMENT_3D('',#32840,#26572,#26573);
#21564=AXIS2_PLACEMENT_3D('',#32841,#26574,#26575);
#21565=AXIS2_PLACEMENT_3D('',#32842,#26576,#26577);
#21566=AXIS2_PLACEMENT_3D('',#32843,#26578,#26579);
#21567=AXIS2_PLACEMENT_3D('',#32844,#26580,#26581);
#21568=AXIS2_PLACEMENT_3D('',#32845,#26582,#26583);
#21569=AXIS2_PLACEMENT_3D('',#32846,#26584,#26585);
#21570=AXIS2_PLACEMENT_3D('',#32847,#26586,#26587);
#21571=AXIS2_PLACEMENT_3D('',#32848,#26588,#26589);
#21572=AXIS2_PLACEMENT_3D('',#32849,#26590,#26591);
#21573=AXIS2_PLACEMENT_3D('',#32850,#26592,#26593);
#21574=AXIS2_PLACEMENT_3D('',#32851,#26594,#26595);
#21575=AXIS2_PLACEMENT_3D('',#32852,#26596,#26597);
#21576=AXIS2_PLACEMENT_3D('',#32853,#26598,#26599);
#21577=AXIS2_PLACEMENT_3D('',#32854,#26600,#26601);
#21578=AXIS2_PLACEMENT_3D('',#32855,#26602,#26603);
#21579=AXIS2_PLACEMENT_3D('',#32856,#26604,#26605);
#21580=AXIS2_PLACEMENT_3D('',#32857,#26606,#26607);
#21581=AXIS2_PLACEMENT_3D('',#32858,#26608,#26609);
#21582=AXIS2_PLACEMENT_3D('',#32859,#26610,#26611);
#21583=AXIS2_PLACEMENT_3D('',#32860,#26612,#26613);
#21584=AXIS2_PLACEMENT_3D('',#32861,#26614,#26615);
#21585=AXIS2_PLACEMENT_3D('',#32862,#26616,#26617);
#21586=AXIS2_PLACEMENT_3D('',#32863,#26618,#26619);
#21587=AXIS2_PLACEMENT_3D('',#32864,#26620,#26621);
#21588=AXIS2_PLACEMENT_3D('',#32865,#26622,#26623);
#21589=AXIS2_PLACEMENT_3D('',#32866,#26624,#26625);
#21590=AXIS2_PLACEMENT_3D('',#32867,#26626,#26627);
#21591=AXIS2_PLACEMENT_3D('',#32868,#26628,#26629);
#21592=AXIS2_PLACEMENT_3D('',#32869,#26630,#26631);
#21593=AXIS2_PLACEMENT_3D('',#32870,#26632,#26633);
#21594=AXIS2_PLACEMENT_3D('',#32871,#26634,#26635);
#21595=AXIS2_PLACEMENT_3D('',#32872,#26636,#26637);
#21596=AXIS2_PLACEMENT_3D('',#32873,#26638,#26639);
#21597=AXIS2_PLACEMENT_3D('',#32874,#26640,#26641);
#21598=AXIS2_PLACEMENT_3D('',#32875,#26642,#26643);
#21599=AXIS2_PLACEMENT_3D('',#32876,#26644,#26645);
#21600=AXIS2_PLACEMENT_3D('',#32877,#26646,#26647);
#21601=AXIS2_PLACEMENT_3D('',#32878,#26648,#26649);
#21602=AXIS2_PLACEMENT_3D('',#32879,#26650,#26651);
#21603=AXIS2_PLACEMENT_3D('',#32880,#26652,#26653);
#21604=AXIS2_PLACEMENT_3D('',#32881,#26654,#26655);
#21605=AXIS2_PLACEMENT_3D('',#32882,#26656,#26657);
#21606=AXIS2_PLACEMENT_3D('',#32883,#26658,#26659);
#21607=AXIS2_PLACEMENT_3D('',#32884,#26660,#26661);
#21608=AXIS2_PLACEMENT_3D('',#32885,#26662,#26663);
#21609=AXIS2_PLACEMENT_3D('',#32886,#26664,#26665);
#21610=AXIS2_PLACEMENT_3D('',#32887,#26666,#26667);
#21611=AXIS2_PLACEMENT_3D('',#32888,#26668,#26669);
#21612=AXIS2_PLACEMENT_3D('',#32889,#26670,#26671);
#21613=AXIS2_PLACEMENT_3D('',#32890,#26672,#26673);
#21614=AXIS2_PLACEMENT_3D('',#32891,#26674,#26675);
#21615=AXIS2_PLACEMENT_3D('',#32892,#26676,#26677);
#21616=AXIS2_PLACEMENT_3D('',#32893,#26678,#26679);
#21617=AXIS2_PLACEMENT_3D('',#32894,#26680,#26681);
#21618=AXIS2_PLACEMENT_3D('',#32895,#26682,#26683);
#21619=AXIS2_PLACEMENT_3D('',#32896,#26684,#26685);
#21620=AXIS2_PLACEMENT_3D('',#32897,#26686,#26687);
#21621=AXIS2_PLACEMENT_3D('',#32898,#26688,#26689);
#21622=AXIS2_PLACEMENT_3D('',#32899,#26690,#26691);
#21623=AXIS2_PLACEMENT_3D('',#32900,#26692,#26693);
#21624=AXIS2_PLACEMENT_3D('',#32901,#26694,#26695);
#21625=AXIS2_PLACEMENT_3D('',#32902,#26696,#26697);
#21626=AXIS2_PLACEMENT_3D('',#32903,#26698,#26699);
#21627=AXIS2_PLACEMENT_3D('',#32904,#26700,#26701);
#21628=AXIS2_PLACEMENT_3D('',#32905,#26702,#26703);
#21629=AXIS2_PLACEMENT_3D('',#32906,#26704,#26705);
#21630=AXIS2_PLACEMENT_3D('',#32907,#26706,#26707);
#21631=AXIS2_PLACEMENT_3D('',#32908,#26708,#26709);
#21632=AXIS2_PLACEMENT_3D('',#32909,#26710,#26711);
#21633=AXIS2_PLACEMENT_3D('',#32910,#26712,#26713);
#21634=AXIS2_PLACEMENT_3D('',#32911,#26714,#26715);
#21635=AXIS2_PLACEMENT_3D('',#32912,#26716,#26717);
#21636=AXIS2_PLACEMENT_3D('',#32913,#26718,#26719);
#21637=AXIS2_PLACEMENT_3D('',#32914,#26720,#26721);
#21638=AXIS2_PLACEMENT_3D('',#32915,#26722,#26723);
#21639=AXIS2_PLACEMENT_3D('',#32916,#26724,#26725);
#21640=AXIS2_PLACEMENT_3D('',#32917,#26726,#26727);
#21641=AXIS2_PLACEMENT_3D('',#32918,#26728,#26729);
#21642=AXIS2_PLACEMENT_3D('',#32919,#26730,#26731);
#21643=AXIS2_PLACEMENT_3D('',#32920,#26732,#26733);
#21644=AXIS2_PLACEMENT_3D('',#32921,#26734,#26735);
#21645=AXIS2_PLACEMENT_3D('',#32922,#26736,#26737);
#21646=AXIS2_PLACEMENT_3D('',#32923,#26738,#26739);
#21647=AXIS2_PLACEMENT_3D('',#32925,#26740,#26741);
#21648=AXIS2_PLACEMENT_3D('',#32926,#26742,#26743);
#21649=AXIS2_PLACEMENT_3D('',#32927,#26744,#26745);
#26104=DIRECTION('axis',(0.,0.,1.));
#26105=DIRECTION('refdir',(1.,0.,0.));
#26106=DIRECTION('center_axis',(6.65798752924967E-17,-1.,1.71022579061586E-31));
#26107=DIRECTION('ref_axis',(-0.345824623417469,-2.30249603002096E-17,0.938299168622762));
#26108=DIRECTION('',(6.65798752924967E-17,-1.,1.71022579061586E-31));
#26109=DIRECTION('center_axis',(6.65798752924967E-17,-1.,1.71022579061586E-31));
#26110=DIRECTION('ref_axis',(-0.345824623433441,-2.3024960301273E-17,0.938299168616875));
#26111=DIRECTION('',(-6.65798752924967E-17,1.,-1.71022579061586E-31));
#26112=DIRECTION('center_axis',(-6.65798752924967E-17,1.,-1.71022579061586E-31));
#26113=DIRECTION('ref_axis',(-0.345824623433441,-2.3024960301273E-17,0.938299168616875));
#26114=DIRECTION('center_axis',(6.65798752924967E-17,-1.,1.71022579061586E-31));
#26115=DIRECTION('ref_axis',(-0.473045086880378,-3.14952828922237E-17,0.881038220384528));
#26116=DIRECTION('',(6.65798752924967E-17,-1.,1.71022579061586E-31));
#26117=DIRECTION('center_axis',(6.65798752924967E-17,-1.,1.71022579061586E-31));
#26118=DIRECTION('ref_axis',(-0.473045086892459,-3.1495282893028E-17,0.881038220378041));
#26119=DIRECTION('',(-6.65798752924967E-17,1.,-1.71022579061586E-31));
#26120=DIRECTION('center_axis',(-6.65798752924967E-17,1.,-1.71022579061586E-31));
#26121=DIRECTION('ref_axis',(-0.473045086892459,-3.1495282893028E-17,0.881038220378041));
#26122=DIRECTION('center_axis',(6.65798752924967E-17,-1.,1.71022579061586E-31));
#26123=DIRECTION('ref_axis',(-0.591058265807973,-3.93525856280941E-17,0.80662886535263));
#26124=DIRECTION('',(6.65798752924967E-17,-1.,1.71022579061586E-31));
#26125=DIRECTION('center_axis',(6.65798752924967E-17,-1.,1.71022579061586E-31));
#26126=DIRECTION('ref_axis',(-0.591058265816149,-3.93525856286384E-17,0.806628865346639));
#26127=DIRECTION('',(-6.65798752924967E-17,1.,-1.71022579061586E-31));
#26128=DIRECTION('center_axis',(-6.65798752924967E-17,1.,-1.71022579061586E-31));
#26129=DIRECTION('ref_axis',(-0.591058265816149,-3.93525856286384E-17,0.806628865346639));
#26130=DIRECTION('center_axis',(6.65798752924967E-17,-1.,1.71022579061586E-31));
#26131=DIRECTION('ref_axis',(-0.697567167910428,-4.64439350476163E-17,0.716519396983379));
#26132=DIRECTION('',(6.65798752924967E-17,-1.,1.71022579061586E-31));
#26133=DIRECTION('center_axis',(6.65798752924967E-17,-1.,1.71022579061586E-31));
#26134=DIRECTION('ref_axis',(-0.697567167914987,-4.64439350479198E-17,0.716519396978941));
#26135=DIRECTION('',(-6.65798752924967E-17,1.,-1.71022579061586E-31));
#26136=DIRECTION('center_axis',(-6.65798752924967E-17,1.,-1.71022579061586E-31));
#26137=DIRECTION('ref_axis',(-0.697567167914987,-4.64439350479198E-17,0.716519396978941));
#26138=DIRECTION('center_axis',(6.65798752924967E-17,-1.,1.71022579061586E-31));
#26139=DIRECTION('ref_axis',(-0.790498718560399,-5.26313061006297E-17,0.61246369358058));
#26140=DIRECTION('',(6.65798752924967E-17,-1.,1.71022579061586E-31));
#26141=DIRECTION('center_axis',(6.65798752924967E-17,-1.,1.71022579061586E-31));
#26142=DIRECTION('ref_axis',(-0.790498718561909,-5.26313061007302E-17,0.612463693578632));
#26143=DIRECTION('',(-6.65798752924967E-17,1.,-1.71022579061586E-31));
#26144=DIRECTION('center_axis',(-6.65798752924967E-17,1.,-1.71022579061586E-31));
#26145=DIRECTION('ref_axis',(-0.790498718561909,-5.26313061007302E-17,0.612463693578632));
#26146=DIRECTION('center_axis',(6.65798752924967E-17,-1.,1.71022579061586E-31));
#26147=DIRECTION('ref_axis',(-0.868044110832557,-5.77942686476178E-17,0.496487081049362));
#26148=DIRECTION('',(6.65798752924967E-17,-1.,1.71022579061586E-31));
#26149=DIRECTION('center_axis',(6.65798752924967E-17,-1.,1.71022579061586E-31));
#26150=DIRECTION('ref_axis',(-0.868044110831822,-5.77942686475688E-17,0.496487081050647));
#26151=DIRECTION('',(-6.65798752924967E-17,1.,-1.71022579061586E-31));
#26152=DIRECTION('center_axis',(-6.65798752924967E-17,1.,-1.71022579061586E-31));
#26153=DIRECTION('ref_axis',(-0.868044110831822,-5.77942686475688E-17,0.496487081050647));
#26154=DIRECTION('center_axis',(6.65798752924967E-17,-1.,1.71022579061586E-31));
#26155=DIRECTION('ref_axis',(-0.928694011872901,-6.18323314953861E-17,0.370846912231201));
#26156=DIRECTION('',(6.65798752924967E-17,-1.,1.71022579061586E-31));
#26157=DIRECTION('center_axis',(6.65798752924967E-17,-1.,1.71022579061586E-31));
#26158=DIRECTION('ref_axis',(-0.9286940118709,-6.18323314952529E-17,0.370846912236213));
#26159=DIRECTION('',(-6.65798752924967E-17,1.,-1.71022579061586E-31));
#26160=DIRECTION('center_axis',(-6.65798752924967E-17,1.,-1.71022579061586E-31));
#26161=DIRECTION('ref_axis',(-0.9286940118709,-6.18323314952529E-17,0.370846912236213));
#26162=DIRECTION('center_axis',(6.65798752924967E-17,-1.,1.71022579061586E-31));
#26163=DIRECTION('ref_axis',(-0.97126794034592,-6.46668983438314E-17,0.237988630098571));
#26164=DIRECTION('',(6.65798752924967E-17,-1.,1.71022579061586E-31));
#26165=DIRECTION('center_axis',(6.65798752924967E-17,-1.,1.71022579061586E-31));
#26166=DIRECTION('ref_axis',(-0.971267940343728,-6.46668983436855E-17,0.237988630107515));
#26167=DIRECTION('',(-6.65798752924967E-17,1.,-1.71022579061586E-31));
#26168=DIRECTION('center_axis',(-6.65798752924967E-17,1.,-1.71022579061586E-31));
#26169=DIRECTION('ref_axis',(-0.971267940343728,-6.46668983436855E-17,0.237988630107515));
#26170=DIRECTION('center_axis',(6.65798752924967E-17,-1.,1.71022579061586E-31));
#26171=DIRECTION('ref_axis',(-0.994937243161013,-6.62427975735207E-17,0.100498169989126));
#26172=DIRECTION('',(6.65798752924967E-17,-1.,1.71022579061586E-31));
#26173=DIRECTION('center_axis',(6.65798752924967E-17,-1.,1.71022579061586E-31));
#26174=DIRECTION('ref_axis',(-0.994937243159722,-6.62427975734348E-17,0.100498170001902));
#26175=DIRECTION('',(-6.65798752924967E-17,1.,-1.71022579061586E-31));
#26176=DIRECTION('center_axis',(-6.65798752924967E-17,1.,-1.71022579061586E-31));
#26177=DIRECTION('ref_axis',(-0.994937243159722,-6.62427975734348E-17,0.100498170001902));
#26178=DIRECTION('center_axis',(6.65798752924967E-17,-1.,1.71022579061586E-31));
#26179=DIRECTION('ref_axis',(-0.999241224262317,-6.65293560985068E-17,-0.0389483726841831));
#26180=DIRECTION('',(6.65798752924967E-17,-1.,1.71022579061586E-31));
#26181=DIRECTION('center_axis',(6.65798752924967E-17,-1.,1.71022579061586E-31));
#26182=DIRECTION('ref_axis',(-0.999241224262949,-6.65293560985489E-17,-0.038948372667972));
#26183=DIRECTION('',(-6.65798752924967E-17,1.,-1.71022579061586E-31));
#26184=DIRECTION('center_axis',(-6.65798752924967E-17,1.,-1.71022579061586E-31));
#26185=DIRECTION('ref_axis',(-0.999241224262949,-6.65293560985489E-17,-0.038948372667972));
#26186=DIRECTION('center_axis',(6.65798752924967E-17,-1.,1.71022579061586E-31));
#26187=DIRECTION('ref_axis',(-0.984096111553401,-6.55209963830564E-17,-0.177636829586311));
#26188=DIRECTION('',(6.65798752924967E-17,-1.,1.71022579061586E-31));
#26189=DIRECTION('center_axis',(6.65798752924967E-17,-1.,1.71022579061586E-31));
#26190=DIRECTION('ref_axis',(-0.984096111556828,-6.55209963832845E-17,-0.177636829567328));
#26191=DIRECTION('',(-6.65798752924967E-17,1.,-1.71022579061586E-31));
#26192=DIRECTION('center_axis',(-6.65798752924967E-17,1.,-1.71022579061586E-31));
#26193=DIRECTION('ref_axis',(-0.984096111556828,-6.55209963832845E-17,-0.177636829567328));
#26194=DIRECTION('center_axis',(6.65798752924967E-17,-1.,1.71022579061586E-31));
#26195=DIRECTION('ref_axis',(-0.949796687425834,-6.32373450020385E-17,-0.312867787659441));
#26196=DIRECTION('',(6.65798752924967E-17,-1.,1.71022579061586E-31));
#26197=DIRECTION('center_axis',(6.65798752924967E-17,-1.,1.71022579061586E-31));
#26198=DIRECTION('ref_axis',(-0.949796687420265,-6.32373450016678E-17,-0.312867787676347));
#26199=DIRECTION('',(-6.65798752924967E-17,1.,-1.71022579061586E-31));
#26200=DIRECTION('center_axis',(-6.65798752924967E-17,1.,-1.71022579061586E-31));
#26201=DIRECTION('ref_axis',(-0.949796687420265,-6.32373450016678E-17,-0.312867787676347));
#26202=DIRECTION('center_axis',(6.65798752924967E-17,-1.,1.71022579061586E-31));
#26203=DIRECTION('ref_axis',(-0.897010551155241,-5.97228506319698E-17,-0.442009130127614));
#26204=DIRECTION('',(6.65798752924967E-17,-1.,1.71022579061586E-31));
#26205=DIRECTION('center_axis',(6.65798752924967E-17,-1.,1.71022579061586E-31));
#26206=DIRECTION('ref_axis',(-0.897010551148803,-5.97228506315411E-17,-0.442009130140681));
#26207=DIRECTION('',(-6.65798752924967E-17,1.,-1.71022579061586E-31));
#26208=DIRECTION('center_axis',(-6.65798752924967E-17,1.,-1.71022579061586E-31));
#26209=DIRECTION('ref_axis',(-0.897010551148803,-5.97228506315411E-17,-0.442009130140681));
#26210=DIRECTION('center_axis',(6.65798752924967E-17,-1.,1.71022579061586E-31));
#26211=DIRECTION('ref_axis',(-0.826765124840791,-5.50459189080855E-17,-0.562547267655786));
#26212=DIRECTION('',(6.65798752924967E-17,-1.,1.71022579061586E-31));
#26213=DIRECTION('center_axis',(6.65798752924967E-17,-1.,1.71022579061586E-31));
#26214=DIRECTION('ref_axis',(-0.826765124834574,-5.50459189076715E-17,-0.562547267664923));
#26215=DIRECTION('',(-6.65798752924967E-17,1.,-1.71022579061586E-31));
#26216=DIRECTION('center_axis',(-6.65798752924967E-17,1.,-1.71022579061586E-31));
#26217=DIRECTION('ref_axis',(-0.826765124834574,-5.50459189076715E-17,-0.562547267664923));
#26218=DIRECTION('center_axis',(6.65798752924967E-17,-1.,1.71022579061586E-31));
#26219=DIRECTION('ref_axis',(-0.740427655802706,-4.929758098646E-17,-0.672136062507071));
#26220=DIRECTION('',(6.65798752924967E-17,-1.,1.71022579061586E-31));
#26221=DIRECTION('center_axis',(6.65798752924967E-17,-1.,1.71022579061586E-31));
#26222=DIRECTION('ref_axis',(-0.740427655797785,-4.92975809861323E-17,-0.672136062512493));
#26223=DIRECTION('',(-6.65798752924967E-17,1.,-1.71022579061586E-31));
#26224=DIRECTION('center_axis',(-6.65798752924967E-17,1.,-1.71022579061586E-31));
#26225=DIRECTION('ref_axis',(-0.740427655797785,-4.92975809861323E-17,-0.672136062512493));
#26226=DIRECTION('center_axis',(6.65798752924967E-17,-1.,1.71022579061586E-31));
#26227=DIRECTION('ref_axis',(-0.639678604668397,-4.25897217261003E-17,-0.768642493445095));
#26228=DIRECTION('',(6.65798752924967E-17,-1.,1.71022579061586E-31));
#26229=DIRECTION('center_axis',(6.65798752924967E-17,-1.,1.71022579061586E-31));
#26230=DIRECTION('ref_axis',(-0.639678604665747,-4.25897217259239E-17,-0.7686424934473));
#26231=DIRECTION('',(-6.65798752924967E-17,1.,-1.71022579061586E-31));
#26232=DIRECTION('center_axis',(-6.65798752924967E-17,1.,-1.71022579061586E-31));
#26233=DIRECTION('ref_axis',(-0.639678604665747,-4.25897217259239E-17,-0.7686424934473));
#26234=DIRECTION('center_axis',(6.65798752924967E-17,-1.,1.71022579061586E-31));
#26235=DIRECTION('ref_axis',(-0.526478937117844,-3.50529019774324E-17,-0.850188172566088));
#26236=DIRECTION('',(6.65798752924967E-17,-1.,1.71022579061586E-31));
#26237=DIRECTION('center_axis',(6.65798752924967E-17,-1.,1.71022579061586E-31));
#26238=DIRECTION('ref_axis',(-0.526478937118264,-3.50529019774604E-17,-0.850188172565828));
#26239=DIRECTION('',(-6.65798752924967E-17,1.,-1.71022579061586E-31));
#26240=DIRECTION('center_axis',(-6.65798752924967E-17,1.,-1.71022579061586E-31));
#26241=DIRECTION('ref_axis',(-0.526478937118264,-3.50529019774604E-17,-0.850188172565828));
#26242=DIRECTION('center_axis',(6.65798752924967E-17,-1.,1.71022579061586E-31));
#26243=DIRECTION('ref_axis',(-0.403031955917209,-2.6833817363859E-17,-0.915185905982795));
#26244=DIRECTION('',(6.65798752924967E-17,-1.,1.71022579061586E-31));
#26245=DIRECTION('center_axis',(6.65798752924967E-17,-1.,1.71022579061586E-31));
#26246=DIRECTION('ref_axis',(-0.403031955921259,-2.68338173641286E-17,-0.915185905981011));
#26247=DIRECTION('',(-6.65798752924967E-17,1.,-1.71022579061586E-31));
#26248=DIRECTION('center_axis',(-6.65798752924967E-17,1.,-1.71022579061586E-31));
#26249=DIRECTION('ref_axis',(-0.403031955921259,-2.68338173641286E-17,-0.915185905981011));
#26250=DIRECTION('center_axis',(6.65798752924967E-17,-1.,1.71022579061586E-31));
#26251=DIRECTION('ref_axis',(-0.2717404161367,-1.80924430183128E-17,-0.962370586748085));
#26252=DIRECTION('',(6.65798752924967E-17,-1.,1.71022579061586E-31));
#26253=DIRECTION('center_axis',(6.65798752924967E-17,-1.,1.71022579061586E-31));
#26254=DIRECTION('ref_axis',(-0.271740416144659,-1.80924430188427E-17,-0.962370586745838));
#26255=DIRECTION('',(-6.65798752924967E-17,1.,-1.71022579061586E-31));
#26256=DIRECTION('center_axis',(-6.65798752924967E-17,1.,-1.71022579061586E-31));
#26257=DIRECTION('ref_axis',(-0.271740416144659,-1.80924430188427E-17,-0.962370586745838));
#26258=DIRECTION('center_axis',(6.65798752924967E-17,-1.,1.71022579061586E-31));
#26259=DIRECTION('ref_axis',(-0.135159758256232,-8.9989198492641E-18,-0.990823818722641));
#26260=DIRECTION('',(6.65798752924967E-17,-1.,1.71022579061586E-31));
#26261=DIRECTION('center_axis',(6.65798752924967E-17,-1.,1.71022579061586E-31));
#26262=DIRECTION('ref_axis',(-0.135159758268076,-8.99891985005266E-18,-0.990823818721025));
#26263=DIRECTION('',(-6.65798752924967E-17,1.,-1.71022579061586E-31));
#26264=DIRECTION('center_axis',(-6.65798752924967E-17,1.,-1.71022579061586E-31));
#26265=DIRECTION('ref_axis',(-0.135159758268076,-8.99891985005266E-18,-0.990823818721025));
#26266=DIRECTION('center_axis',(6.65798752924967E-17,-1.,1.71022579061586E-31));
#26267=DIRECTION('ref_axis',(0.00405163057674682,2.69757058530899E-19,-0.99999179211115));
#26268=DIRECTION('',(6.65798752924967E-17,-1.,1.71022579061586E-31));
#26269=DIRECTION('center_axis',(6.65798752924967E-17,-1.,1.71022579061586E-31));
#26270=DIRECTION('ref_axis',(0.00405163056134247,2.69757057505279E-19,-0.999991792111212));
#26271=DIRECTION('',(-6.65798752924967E-17,1.,-1.71022579061586E-31));
#26272=DIRECTION('center_axis',(-6.65798752924967E-17,1.,-1.71022579061586E-31));
#26273=DIRECTION('ref_axis',(0.00405163056134247,2.69757057505279E-19,-0.999991792111212));
#26274=DIRECTION('center_axis',(6.65798752924967E-17,-1.,1.71022579061586E-31));
#26275=DIRECTION('ref_axis',(0.143184159029212,9.53318345202578E-18,-0.98969606274002));
#26276=DIRECTION('',(6.65798752924967E-17,-1.,1.71022579061586E-31));
#26277=DIRECTION('center_axis',(6.65798752924967E-17,-1.,1.71022579061586E-31));
#26278=DIRECTION('ref_axis',(0.143184159010847,9.53318345080304E-18,-0.989696062742677));
#26279=DIRECTION('',(-6.65798752924967E-17,1.,-1.71022579061586E-31));
#26280=DIRECTION('center_axis',(-6.65798752924967E-17,1.,-1.71022579061586E-31));
#26281=DIRECTION('ref_axis',(0.143184159010847,9.53318345080304E-18,-0.989696062742677));
#26282=DIRECTION('center_axis',(6.65798752924967E-17,-1.,1.71022579061586E-31));
#26283=DIRECTION('ref_axis',(0.27952977069574,1.86110572734624E-17,-0.960137025270241));
#26284=DIRECTION('',(6.65798752924967E-17,-1.,1.71022579061586E-31));
#26285=DIRECTION('center_axis',(6.65798752924967E-17,-1.,1.71022579061586E-31));
#26286=DIRECTION('ref_axis',(0.279529770713557,1.86110572746487E-17,-0.960137025265054));
#26287=DIRECTION('',(-6.65798752924967E-17,1.,-1.71022579061586E-31));
#26288=DIRECTION('center_axis',(-6.65798752924967E-17,1.,-1.71022579061586E-31));
#26289=DIRECTION('ref_axis',(0.279529770713557,1.86110572746487E-17,-0.960137025265054));
#26290=DIRECTION('center_axis',(6.65798752924967E-17,-1.,1.71022579061586E-31));
#26291=DIRECTION('ref_axis',(0.410434653336076,2.73266880348349E-17,-0.911890012743256));
#26292=DIRECTION('',(6.65798752924967E-17,-1.,1.71022579061586E-31));
#26293=DIRECTION('center_axis',(6.65798752924967E-17,-1.,1.71022579061586E-31));
#26294=DIRECTION('ref_axis',(0.410434653350123,2.73266880357702E-17,-0.911890012736933));
#26295=DIRECTION('',(-6.65798752924967E-17,1.,-1.71022579061586E-31));
#26296=DIRECTION('center_axis',(-6.65798752924967E-17,1.,-1.71022579061586E-31));
#26297=DIRECTION('ref_axis',(0.410434653350123,2.73266880357702E-17,-0.911890012736933));
#26298=DIRECTION('center_axis',(6.65798752924967E-17,-1.,1.71022579061586E-31));
#26299=DIRECTION('ref_axis',(0.533350892311725,3.55104358972563E-17,-0.845894098377738));
#26300=DIRECTION('',(6.65798752924967E-17,-1.,1.71022579061586E-31));
#26301=DIRECTION('center_axis',(6.65798752924967E-17,-1.,1.71022579061586E-31));
#26302=DIRECTION('ref_axis',(0.533350892321836,3.55104358979295E-17,-0.845894098371363));
#26303=DIRECTION('',(-6.65798752924967E-17,1.,-1.71022579061586E-31));
#26304=DIRECTION('center_axis',(-6.65798752924967E-17,1.,-1.71022579061586E-31));
#26305=DIRECTION('ref_axis',(0.533350892321836,3.55104358979295E-17,-0.845894098371363));
#26306=DIRECTION('center_axis',(6.65798752924967E-17,-1.,1.71022579061586E-31));
#26307=DIRECTION('ref_axis',(0.645886062846174,4.30030135174598E-17,-0.763433817577574));
#26308=DIRECTION('',(6.65798752924967E-17,-1.,1.71022579061586E-31));
#26309=DIRECTION('center_axis',(6.65798752924967E-17,-1.,1.71022579061586E-31));
#26310=DIRECTION('ref_axis',(0.645886062852486,4.30030135178801E-17,-0.763433817572233));
#26311=DIRECTION('',(-6.65798752924967E-17,1.,-1.71022579061586E-31));
#26312=DIRECTION('center_axis',(-6.65798752924967E-17,1.,-1.71022579061586E-31));
#26313=DIRECTION('ref_axis',(0.645886062852486,4.30030135178801E-17,-0.763433817572233));
#26314=DIRECTION('center_axis',(6.65798752924967E-17,-1.,1.71022579061586E-31));
#26315=DIRECTION('ref_axis',(0.745849795851828,4.96585863947487E-17,-0.666114165911359));
#26316=DIRECTION('',(6.65798752924967E-17,-1.,1.71022579061586E-31));
#26317=DIRECTION('center_axis',(6.65798752924967E-17,-1.,1.71022579061586E-31));
#26318=DIRECTION('ref_axis',(0.745849795854776,4.9658586394945E-17,-0.66611416590806));
#26319=DIRECTION('',(-6.65798752924967E-17,1.,-1.71022579061586E-31));
#26320=DIRECTION('center_axis',(-6.65798752924967E-17,1.,-1.71022579061586E-31));
#26321=DIRECTION('ref_axis',(0.745849795854776,4.9658586394945E-17,-0.66611416590806));
#26322=DIRECTION('center_axis',(6.65798752924967E-17,-1.,1.71022579061586E-31));
#26323=DIRECTION('ref_axis',(0.831296410972796,5.53476113736688E-17,-0.555829359699313));
#26324=DIRECTION('',(6.65798752924967E-17,-1.,1.71022579061586E-31));
#26325=DIRECTION('center_axis',(6.65798752924967E-17,-1.,1.71022579061586E-31));
#26326=DIRECTION('ref_axis',(0.83129641097307,5.5347611373687E-17,-0.555829359698903));
#26327=DIRECTION('',(-6.65798752924967E-17,1.,-1.71022579061586E-31));
#26328=DIRECTION('center_axis',(-6.65798752924967E-17,1.,-1.71022579061586E-31));
#26329=DIRECTION('ref_axis',(0.83129641097307,5.5347611373687E-17,-0.555829359698903));
#26330=DIRECTION('center_axis',(6.65798752924967E-17,-1.,1.71022579061586E-31));
#26331=DIRECTION('ref_axis',(0.900562787039831,5.99593580541751E-17,-0.434725967247245));
#26332=DIRECTION('',(6.65798752924967E-17,-1.,1.71022579061586E-31));
#26333=DIRECTION('center_axis',(6.65798752924967E-17,-1.,1.71022579061586E-31));
#26334=DIRECTION('ref_axis',(0.900562787038332,5.99593580540753E-17,-0.434725967250349));
#26335=DIRECTION('',(-6.65798752924967E-17,1.,-1.71022579061586E-31));
#26336=DIRECTION('center_axis',(-6.65798752924967E-17,1.,-1.71022579061586E-31));
#26337=DIRECTION('ref_axis',(0.900562787038332,5.99593580540753E-17,-0.434725967250349));
#26338=DIRECTION('center_axis',(6.65798752924967E-17,-1.,1.71022579061586E-31));
#26339=DIRECTION('ref_axis',(0.952300732832122,6.34040640329159E-17,-0.305161128336168));
#26340=DIRECTION('',(6.65798752924967E-17,-1.,1.71022579061586E-31));
#26341=DIRECTION('center_axis',(6.65798752924967E-17,-1.,1.71022579061586E-31));
#26342=DIRECTION('ref_axis',(0.952300732829888,6.34040640327671E-17,-0.30516112834314));
#26343=DIRECTION('',(-6.65798752924967E-17,1.,-1.71022579061586E-31));
#26344=DIRECTION('center_axis',(-6.65798752924967E-17,1.,-1.71022579061586E-31));
#26345=DIRECTION('ref_axis',(0.952300732829888,6.34040640327671E-17,-0.30516112834314));
#26346=DIRECTION('center_axis',(6.65798752924967E-17,-1.,1.71022579061586E-31));
#26347=DIRECTION('ref_axis',(0.985503228085865,6.56146820263098E-17,-0.169656675177667));
#26348=DIRECTION('',(6.65798752924967E-17,-1.,1.71022579061586E-31));
#26349=DIRECTION('center_axis',(6.65798752924967E-17,-1.,1.71022579061586E-31));
#26350=DIRECTION('ref_axis',(0.985503228083989,6.56146820261849E-17,-0.169656675188558));
#26351=DIRECTION('',(-6.65798752924967E-17,1.,-1.71022579061586E-31));
#26352=DIRECTION('center_axis',(-6.65798752924967E-17,1.,-1.71022579061586E-31));
#26353=DIRECTION('ref_axis',(0.985503228083989,6.56146820261849E-17,-0.169656675188558));
#26354=DIRECTION('center_axis',(6.65798752924967E-17,-1.,1.71022579061586E-31));
#26355=DIRECTION('ref_axis',(0.999524023998223,6.65481848696562E-17,-0.0308500478184399));
#26356=DIRECTION('',(6.65798752924967E-17,-1.,1.71022579061586E-31));
#26357=DIRECTION('center_axis',(6.65798752924967E-17,-1.,1.71022579061586E-31));
#26358=DIRECTION('ref_axis',(0.999524023997774,6.65481848696262E-17,-0.0308500478330001));
#26359=DIRECTION('',(-6.65798752924967E-17,1.,-1.71022579061586E-31));
#26360=DIRECTION('center_axis',(-6.65798752924967E-17,1.,-1.71022579061586E-31));
#26361=DIRECTION('ref_axis',(0.999524023997774,6.65481848696262E-17,-0.0308500478330001));
#26362=DIRECTION('center_axis',(6.65798752924967E-17,-1.,1.71022579061586E-31));
#26363=DIRECTION('ref_axis',(0.994090221725182,6.6186402991953E-17,0.108557040630164));
#26364=DIRECTION('',(6.65798752924967E-17,-1.,1.71022579061586E-31));
#26365=DIRECTION('center_axis',(6.65798752924967E-17,-1.,1.71022579061586E-31));
#26366=DIRECTION('ref_axis',(0.994090221727114,6.61864029920817E-17,0.108557040612469));
#26367=DIRECTION('',(-6.65798752924967E-17,1.,-1.71022579061586E-31));
#26368=DIRECTION('center_axis',(-6.65798752924967E-17,1.,-1.71022579061586E-31));
#26369=DIRECTION('ref_axis',(0.994090221727114,6.61864029920817E-17,0.108557040612469));
#26370=DIRECTION('center_axis',(6.65798752924967E-17,-1.,1.71022579061586E-31));
#26371=DIRECTION('ref_axis',(0.969307584047127,6.4536378065929E-17,0.245851189764706));
#26372=DIRECTION('',(6.65798752924967E-17,-1.,1.71022579061586E-31));
#26373=DIRECTION('center_axis',(6.65798752924967E-17,-1.,1.71022579061586E-31));
#26374=DIRECTION('ref_axis',(0.969307584042385,6.45363780656133E-17,0.245851189783404));
#26375=DIRECTION('',(-6.65798752924967E-17,1.,-1.71022579061586E-31));
#26376=DIRECTION('center_axis',(-6.65798752924967E-17,1.,-1.71022579061586E-31));
#26377=DIRECTION('ref_axis',(0.969307584042385,6.45363780656133E-17,0.245851189783404));
#26378=DIRECTION('center_axis',(6.65798752924967E-17,-1.,1.71022579061586E-31));
#26379=DIRECTION('ref_axis',(0.925658476816631,6.16302259498938E-17,0.37836012514206));
#26380=DIRECTION('',(6.65798752924967E-17,-1.,1.71022579061586E-31));
#26381=DIRECTION('center_axis',(6.65798752924967E-17,-1.,1.71022579061586E-31));
#26382=DIRECTION('ref_axis',(0.925658476810492,6.16302259494851E-17,0.378360125157078));
#26383=DIRECTION('',(-6.65798752924967E-17,1.,-1.71022579061586E-31));
#26384=DIRECTION('center_axis',(-6.65798752924967E-17,1.,-1.71022579061586E-31));
#26385=DIRECTION('ref_axis',(0.925658476810492,6.16302259494851E-17,0.378360125157078));
#26386=DIRECTION('center_axis',(6.65798752924967E-17,-1.,1.71022579061586E-31));
#26387=DIRECTION('ref_axis',(0.86399248025581,5.75245115890868E-17,0.503504711061788));
#26388=DIRECTION('',(6.65798752924967E-17,-1.,1.71022579061586E-31));
#26389=DIRECTION('center_axis',(6.65798752924967E-17,-1.,1.71022579061586E-31));
#26390=DIRECTION('ref_axis',(0.863992480249344,5.75245115886563E-17,0.503504711072882));
#26391=DIRECTION('',(-6.65798752924967E-17,1.,-1.71022579061586E-31));
#26392=DIRECTION('center_axis',(-6.65798752924967E-17,1.,-1.71022579061586E-31));
#26393=DIRECTION('ref_axis',(0.863992480249344,5.75245115886563E-17,0.503504711072882));
#26394=DIRECTION('center_axis',(6.65798752924967E-17,-1.,1.71022579061586E-31));
#26395=DIRECTION('ref_axis',(0.785509852843689,5.22991480433604E-17,0.618849150508818));
#26396=DIRECTION('',(6.65798752924967E-17,-1.,1.71022579061586E-31));
#26397=DIRECTION('center_axis',(6.65798752924967E-17,-1.,1.71022579061586E-31));
#26398=DIRECTION('ref_axis',(0.78550985283799,5.22991480429809E-17,0.618849150516052));
#26399=DIRECTION('',(-6.65798752924967E-17,1.,-1.71022579061586E-31));
#26400=DIRECTION('center_axis',(-6.65798752924967E-17,1.,-1.71022579061586E-31));
#26401=DIRECTION('ref_axis',(0.78550985283799,5.22991480429809E-17,0.618849150516052));
#26402=DIRECTION('center_axis',(6.65798752924967E-17,-1.,1.71022579061586E-31));
#26403=DIRECTION('ref_axis',(0.691738169650181,4.60558410703691E-17,0.72214839517167));
#26404=DIRECTION('',(6.65798752924967E-17,-1.,1.71022579061586E-31));
#26405=DIRECTION('center_axis',(6.65798752924967E-17,-1.,1.71022579061586E-31));
#26406=DIRECTION('ref_axis',(0.691738169646283,4.60558410701096E-17,0.722148395175403));
#26407=DIRECTION('',(-6.65798752924967E-17,1.,-1.71022579061586E-31));
#26408=DIRECTION('center_axis',(-6.65798752924967E-17,1.,-1.71022579061586E-31));
#26409=DIRECTION('ref_axis',(0.691738169646283,4.60558410701096E-17,0.722148395175403));
#26410=DIRECTION('center_axis',(6.65798752924967E-17,-1.,1.71022579061586E-31));
#26411=DIRECTION('ref_axis',(0.584502589824937,3.89161095386858E-17,0.811391842754129));
#26412=DIRECTION('',(6.65798752924967E-17,-1.,1.71022579061586E-31));
#26413=DIRECTION('center_axis',(6.65798752924967E-17,-1.,1.71022579061586E-31));
#26414=DIRECTION('ref_axis',(0.584502589823736,3.89161095386059E-17,0.811391842754994));
#26415=DIRECTION('',(-6.65798752924967E-17,1.,-1.71022579061586E-31));
#26416=DIRECTION('center_axis',(-6.65798752924967E-17,1.,-1.71022579061586E-31));
#26417=DIRECTION('ref_axis',(0.584502589823736,3.89161095386059E-17,0.811391842754994));
#26418=DIRECTION('center_axis',(6.65798752924967E-17,-1.,1.71022579061586E-31));
#26419=DIRECTION('ref_axis',(0.465890331950592,3.10189202012505E-17,0.884842471061921));
#26420=DIRECTION('',(6.65798752924967E-17,-1.,1.71022579061586E-31));
#26421=DIRECTION('center_axis',(6.65798752924967E-17,-1.,1.71022579061586E-31));
#26422=DIRECTION('ref_axis',(0.465890331952774,3.10189202013957E-17,0.884842471060773));
#26423=DIRECTION('',(-6.65798752924967E-17,1.,-1.71022579061586E-31));
#26424=DIRECTION('center_axis',(-6.65798752924967E-17,1.,-1.71022579061586E-31));
#26425=DIRECTION('ref_axis',(0.465890331952774,3.10189202013957E-17,0.884842471060773));
#26426=DIRECTION('center_axis',(6.65798752924967E-17,-1.,1.71022579061586E-31));
#26427=DIRECTION('ref_axis',(0.338210048707227,2.25179828655966E-17,0.941070647163886));
#26428=DIRECTION('',(6.65798752924967E-17,-1.,1.71022579061586E-31));
#26429=DIRECTION('center_axis',(6.65798752924967E-17,-1.,1.71022579061586E-31));
#26430=DIRECTION('ref_axis',(0.338210048713215,2.25179828659953E-17,0.941070647161734));
#26431=DIRECTION('',(-6.65798752924967E-17,1.,-1.71022579061586E-31));
#26432=DIRECTION('center_axis',(-6.65798752924967E-17,1.,-1.71022579061586E-31));
#26433=DIRECTION('ref_axis',(0.338210048713215,2.25179828659953E-17,0.941070647161734));
#26434=DIRECTION('center_axis',(6.65798752924967E-17,-1.,1.71022579061586E-31));
#26435=DIRECTION('ref_axis',(0.203946891574005,1.35787586072898E-17,0.978981953570801));
#26436=DIRECTION('',(6.65798752924967E-17,-1.,1.71022579061586E-31));
#26437=DIRECTION('center_axis',(6.65798752924967E-17,-1.,1.71022579061586E-31));
#26438=DIRECTION('ref_axis',(0.203946891583929,1.35787586079505E-17,0.978981953568733));
#26439=DIRECTION('',(-6.65798752924967E-17,1.,-1.71022579061586E-31));
#26440=DIRECTION('center_axis',(-6.65798752924967E-17,1.,-1.71022579061586E-31));
#26441=DIRECTION('ref_axis',(0.203946891583929,1.35787586079505E-17,0.978981953568733));
#26442=DIRECTION('center_axis',(6.65798752924967E-17,-1.,1.71022579061586E-31));
#26443=DIRECTION('ref_axis',(0.0657141401824452,4.37523925830102E-18,0.997838489826927));
#26444=DIRECTION('',(6.65798752924967E-17,-1.,1.71022579061586E-31));
#26445=DIRECTION('center_axis',(6.65798752924967E-17,-1.,1.71022579061586E-31));
#26446=DIRECTION('ref_axis',(0.0657141401961282,4.37523925921203E-18,0.997838489826026));
#26447=DIRECTION('',(-6.65798752924967E-17,1.,-1.71022579061586E-31));
#26448=DIRECTION('center_axis',(-6.65798752924967E-17,1.,-1.71022579061586E-31));
#26449=DIRECTION('ref_axis',(0.0657141401961282,4.37523925921203E-18,0.997838489826026));
#26450=DIRECTION('center_axis',(6.65798752924967E-17,-1.,1.71022579061586E-31));
#26451=DIRECTION('ref_axis',(-0.0737976621990395,-4.91343914608968E-18,
0.997273234903031));
#26452=DIRECTION('',(6.65798752924967E-17,-1.,1.71022579061586E-31));
#26453=DIRECTION('center_axis',(6.65798752924967E-17,-1.,1.71022579061586E-31));
#26454=DIRECTION('ref_axis',(-0.073797662182064,-4.91343914495945E-18,0.997273234904287));
#26455=DIRECTION('',(-6.65798752924967E-17,1.,-1.71022579061586E-31));
#26456=DIRECTION('center_axis',(-6.65798752924967E-17,1.,-1.71022579061586E-31));
#26457=DIRECTION('ref_axis',(-0.073797662182064,-4.91343914495945E-18,0.997273234904287));
#26458=DIRECTION('center_axis',(-6.65798752924967E-17,1.,-1.71022579061586E-31));
#26459=DIRECTION('ref_axis',(-0.211873077029416,-1.41064830464559E-17,0.97729719084324));
#26460=DIRECTION('center_axis',(-6.65798752924967E-17,1.,-1.71022579061586E-31));
#26461=DIRECTION('ref_axis',(-0.211873077029416,-1.41064830464559E-17,0.97729719084324));
#26462=DIRECTION('center_axis',(6.65798752924967E-17,-1.,1.71022579061586E-31));
#26463=DIRECTION('ref_axis',(-0.211873077029416,-1.41064830464559E-17,0.977297190843239));
#26464=DIRECTION('center_axis',(-6.65798752924967E-17,1.,-1.71022579061586E-31));
#26465=DIRECTION('ref_axis',(-0.211873077029416,-1.41064830464559E-17,0.97729719084324));
#26466=DIRECTION('center_axis',(-6.65798752924967E-17,1.,-1.71022579061586E-31));
#26467=DIRECTION('ref_axis',(-0.211873077029416,-1.41064830464559E-17,0.97729719084324));
#26468=DIRECTION('center_axis',(-6.65798752924967E-17,1.,-1.71022579061586E-31));
#26469=DIRECTION('ref_axis',(-0.211873077029416,-1.41064830464559E-17,0.97729719084324));
#26470=DIRECTION('center_axis',(-6.65798752924967E-17,1.,-1.71022579061586E-31));
#26471=DIRECTION('ref_axis',(-0.211873077029416,-1.41064830464559E-17,0.97729719084324));
#26472=DIRECTION('center_axis',(-6.65798752924967E-17,1.,-1.71022579061586E-31));
#26473=DIRECTION('ref_axis',(-0.211873077029416,-1.41064830464559E-17,0.97729719084324));
#26474=DIRECTION('center_axis',(-6.65798752924967E-17,1.,-1.71022579061586E-31));
#26475=DIRECTION('ref_axis',(-0.211873077029416,-1.41064830464559E-17,0.97729719084324));
#26476=DIRECTION('center_axis',(-6.65798752924967E-17,1.,-1.71022579061586E-31));
#26477=DIRECTION('ref_axis',(-0.211873077029416,-1.41064830464559E-17,0.97729719084324));
#26478=DIRECTION('center_axis',(-6.65798752924967E-17,1.,-1.71022579061586E-31));
#26479=DIRECTION('ref_axis',(-0.211873077029416,-1.41064830464559E-17,0.97729719084324));
#26480=DIRECTION('center_axis',(-6.65798752924967E-17,1.,-1.71022579061586E-31));
#26481=DIRECTION('ref_axis',(-0.211873077029416,-1.41064830464559E-17,0.97729719084324));
#26482=DIRECTION('center_axis',(-6.65798752924967E-17,1.,-1.71022579061586E-31));
#26483=DIRECTION('ref_axis',(-0.211873077029416,-1.41064830464559E-17,0.97729719084324));
#26484=DIRECTION('center_axis',(-6.65798752924967E-17,1.,-1.71022579061586E-31));
#26485=DIRECTION('ref_axis',(-0.211873077029416,-1.41064830464559E-17,0.97729719084324));
#26486=DIRECTION('center_axis',(-6.65798752924967E-17,1.,-1.71022579061586E-31));
#26487=DIRECTION('ref_axis',(-0.211873077029416,-1.41064830464559E-17,0.97729719084324));
#26488=DIRECTION('center_axis',(-6.65798752924967E-17,1.,-1.71022579061586E-31));
#26489=DIRECTION('ref_axis',(-0.211873077029416,-1.41064830464559E-17,0.97729719084324));
#26490=DIRECTION('center_axis',(-6.65798752924967E-17,1.,-1.71022579061586E-31));
#26491=DIRECTION('ref_axis',(-0.211873077029416,-1.41064830464559E-17,0.97729719084324));
#26492=DIRECTION('center_axis',(-6.65798752924967E-17,1.,-1.71022579061586E-31));
#26493=DIRECTION('ref_axis',(-0.211873077029416,-1.41064830464559E-17,0.97729719084324));
#26494=DIRECTION('center_axis',(-6.65798752924967E-17,1.,-1.71022579061586E-31));
#26495=DIRECTION('ref_axis',(-0.211873077029416,-1.41064830464559E-17,0.97729719084324));
#26496=DIRECTION('center_axis',(-6.65798752924967E-17,1.,-1.71022579061586E-31));
#26497=DIRECTION('ref_axis',(-0.211873077029416,-1.41064830464559E-17,0.97729719084324));
#26498=DIRECTION('center_axis',(-6.65798752924967E-17,1.,-1.71022579061586E-31));
#26499=DIRECTION('ref_axis',(-0.211873077029416,-1.41064830464559E-17,0.97729719084324));
#26500=DIRECTION('center_axis',(-6.65798752924967E-17,1.,-1.71022579061586E-31));
#26501=DIRECTION('ref_axis',(-0.211873077029416,-1.41064830464559E-17,0.97729719084324));
#26502=DIRECTION('center_axis',(-6.65798752924967E-17,1.,-1.71022579061586E-31));
#26503=DIRECTION('ref_axis',(-0.211873077029416,-1.41064830464559E-17,0.97729719084324));
#26504=DIRECTION('center_axis',(-6.65798752924967E-17,1.,-1.71022579061586E-31));
#26505=DIRECTION('ref_axis',(-0.211873077029416,-1.41064830464559E-17,0.97729719084324));
#26506=DIRECTION('center_axis',(-6.65798752924967E-17,1.,-1.71022579061586E-31));
#26507=DIRECTION('ref_axis',(-0.211873077029416,-1.41064830464559E-17,0.97729719084324));
#26508=DIRECTION('center_axis',(-6.65798752924967E-17,1.,-1.71022579061586E-31));
#26509=DIRECTION('ref_axis',(-0.211873077029416,-1.41064830464559E-17,0.97729719084324));
#26510=DIRECTION('center_axis',(-6.65798752924967E-17,1.,-1.71022579061586E-31));
#26511=DIRECTION('ref_axis',(-0.211873077029416,-1.41064830464559E-17,0.97729719084324));
#26512=DIRECTION('center_axis',(-6.65798752924967E-17,1.,-1.71022579061586E-31));
#26513=DIRECTION('ref_axis',(-0.211873077029416,-1.41064830464559E-17,0.97729719084324));
#26514=DIRECTION('center_axis',(-6.65798752924967E-17,1.,-1.71022579061586E-31));
#26515=DIRECTION('ref_axis',(-0.211873077029416,-1.41064830464559E-17,0.97729719084324));
#26516=DIRECTION('center_axis',(-6.65798752924967E-17,1.,-1.71022579061586E-31));
#26517=DIRECTION('ref_axis',(-0.211873077029416,-1.41064830464559E-17,0.97729719084324));
#26518=DIRECTION('center_axis',(-6.65798752924967E-17,1.,-1.71022579061586E-31));
#26519=DIRECTION('ref_axis',(-0.211873077029416,-1.41064830464559E-17,0.97729719084324));
#26520=DIRECTION('center_axis',(-6.65798752924967E-17,1.,-1.71022579061586E-31));
#26521=DIRECTION('ref_axis',(-0.211873077029416,-1.41064830464559E-17,0.97729719084324));
#26522=DIRECTION('center_axis',(-6.65798752924967E-17,1.,-1.71022579061586E-31));
#26523=DIRECTION('ref_axis',(-0.211873077029416,-1.41064830464559E-17,0.97729719084324));
#26524=DIRECTION('center_axis',(-6.65798752924967E-17,1.,-1.71022579061586E-31));
#26525=DIRECTION('ref_axis',(-0.211873077029416,-1.41064830464559E-17,0.97729719084324));
#26526=DIRECTION('center_axis',(-6.65798752924967E-17,1.,-1.71022579061586E-31));
#26527=DIRECTION('ref_axis',(-0.211873077029416,-1.41064830464559E-17,0.97729719084324));
#26528=DIRECTION('center_axis',(-6.65798752924967E-17,1.,-1.71022579061586E-31));
#26529=DIRECTION('ref_axis',(-0.211873077029416,-1.41064830464559E-17,0.97729719084324));
#26530=DIRECTION('center_axis',(-6.65798752924967E-17,1.,-1.71022579061586E-31));
#26531=DIRECTION('ref_axis',(-0.211873077029416,-1.41064830464559E-17,0.97729719084324));
#26532=DIRECTION('center_axis',(-6.65798752924967E-17,1.,-1.71022579061586E-31));
#26533=DIRECTION('ref_axis',(-0.211873077029416,-1.41064830464559E-17,0.97729719084324));
#26534=DIRECTION('center_axis',(-6.65798752924967E-17,1.,-1.71022579061586E-31));
#26535=DIRECTION('ref_axis',(-0.211873077029416,-1.41064830464559E-17,0.97729719084324));
#26536=DIRECTION('center_axis',(-6.65798752924967E-17,1.,-1.71022579061586E-31));
#26537=DIRECTION('ref_axis',(-0.211873077029416,-1.41064830464559E-17,0.97729719084324));
#26538=DIRECTION('center_axis',(-6.65798752924967E-17,1.,-1.71022579061586E-31));
#26539=DIRECTION('ref_axis',(-0.211873077029416,-1.41064830464559E-17,0.97729719084324));
#26540=DIRECTION('center_axis',(-6.65798752924967E-17,1.,-1.71022579061586E-31));
#26541=DIRECTION('ref_axis',(-0.211873077029416,-1.41064830464559E-17,0.97729719084324));
#26542=DIRECTION('center_axis',(-6.65798752924967E-17,1.,-1.71022579061586E-31));
#26543=DIRECTION('ref_axis',(-0.211873077029416,-1.41064830464559E-17,0.97729719084324));
#26544=DIRECTION('center_axis',(-6.65798752924967E-17,1.,-1.71022579061586E-31));
#26545=DIRECTION('ref_axis',(-0.211873077029416,-1.41064830464559E-17,0.97729719084324));
#26546=DIRECTION('center_axis',(-6.65798752924967E-17,1.,-1.71022579061586E-31));
#26547=DIRECTION('ref_axis',(-0.211873077029416,-1.41064830464559E-17,0.97729719084324));
#26548=DIRECTION('center_axis',(-6.65798752924967E-17,1.,-1.71022579061586E-31));
#26549=DIRECTION('ref_axis',(-0.211873077029416,-1.41064830464559E-17,0.97729719084324));
#26550=DIRECTION('center_axis',(-6.65798752924967E-17,1.,-1.71022579061586E-31));
#26551=DIRECTION('ref_axis',(-0.211873077029416,-1.41064830464559E-17,0.97729719084324));
#26552=DIRECTION('center_axis',(6.65798752924967E-17,-1.,1.71022579061586E-31));
#26553=DIRECTION('ref_axis',(0.211873077029416,1.41064830464559E-17,-0.977297190843239));
#26554=DIRECTION('center_axis',(-6.65798752924967E-17,1.,-1.71022579061586E-31));
#26555=DIRECTION('ref_axis',(-0.211873077029416,-1.41064830464559E-17,0.977297190843239));
#26556=DIRECTION('center_axis',(-6.65798752924967E-17,1.,-1.71022579061586E-31));
#26557=DIRECTION('ref_axis',(-0.211873077029416,-1.41064830464559E-17,0.97729719084324));
#26558=DIRECTION('',(-6.65798752924967E-17,1.,-1.71022579061586E-31));
#26559=DIRECTION('center_axis',(-6.65798752924967E-17,1.,-1.71022579061586E-31));
#26560=DIRECTION('ref_axis',(-0.211873077029416,-1.41064830464559E-17,0.977297190843239));
#26561=DIRECTION('',(6.65798752924967E-17,-1.,1.71022579061586E-31));
#26562=DIRECTION('center_axis',(-6.65798752924967E-17,1.,-1.71022579061586E-31));
#26563=DIRECTION('ref_axis',(-0.211873077029416,-1.41064830464559E-17,0.97729719084324));
#26564=DIRECTION('center_axis',(-6.65798752924967E-17,1.,-1.71022579061586E-31));
#26565=DIRECTION('ref_axis',(-0.211873077029416,-1.41064830464559E-17,0.977297190843239));
#26566=DIRECTION('center_axis',(-6.65798752924967E-17,1.,-1.71022579061586E-31));
#26567=DIRECTION('ref_axis',(-0.211873077029416,-1.41064830464559E-17,0.97729719084324));
#26568=DIRECTION('center_axis',(-6.65798752924967E-17,1.,-1.71022579061586E-31));
#26569=DIRECTION('ref_axis',(-0.211873077029416,-1.41064830464559E-17,0.977297190843239));
#26570=DIRECTION('center_axis',(-6.65798752924967E-17,1.,-1.71022579061586E-31));
#26571=DIRECTION('ref_axis',(-0.211873077029416,-1.41064830464559E-17,0.97729719084324));
#26572=DIRECTION('center_axis',(-6.65798752924967E-17,1.,-1.71022579061586E-31));
#26573=DIRECTION('ref_axis',(-0.211873077029416,-1.41064830464559E-17,0.977297190843239));
#26574=DIRECTION('center_axis',(-6.65798752924967E-17,1.,-1.71022579061586E-31));
#26575=DIRECTION('ref_axis',(-0.211873077029416,-1.41064830464559E-17,0.97729719084324));
#26576=DIRECTION('center_axis',(-6.65798752924967E-17,1.,-1.71022579061586E-31));
#26577=DIRECTION('ref_axis',(-0.211873077029416,-1.41064830464559E-17,0.977297190843239));
#26578=DIRECTION('center_axis',(-6.65798752924967E-17,1.,-1.71022579061586E-31));
#26579=DIRECTION('ref_axis',(-0.211873077029416,-1.41064830464559E-17,0.97729719084324));
#26580=DIRECTION('center_axis',(-6.65798752924967E-17,1.,-1.71022579061586E-31));
#26581=DIRECTION('ref_axis',(-0.211873077029416,-1.41064830464559E-17,0.977297190843239));
#26582=DIRECTION('center_axis',(-6.65798752924967E-17,1.,-1.71022579061586E-31));
#26583=DIRECTION('ref_axis',(-0.211873077029416,-1.41064830464559E-17,0.97729719084324));
#26584=DIRECTION('center_axis',(-6.65798752924967E-17,1.,-1.71022579061586E-31));
#26585=DIRECTION('ref_axis',(-0.211873077029416,-1.41064830464559E-17,0.977297190843239));
#26586=DIRECTION('center_axis',(-6.65798752924967E-17,1.,-1.71022579061586E-31));
#26587=DIRECTION('ref_axis',(-0.211873077029416,-1.41064830464559E-17,0.97729719084324));
#26588=DIRECTION('center_axis',(-6.65798752924967E-17,1.,-1.71022579061586E-31));
#26589=DIRECTION('ref_axis',(-0.211873077029416,-1.41064830464559E-17,0.977297190843239));
#26590=DIRECTION('center_axis',(-6.65798752924967E-17,1.,-1.71022579061586E-31));
#26591=DIRECTION('ref_axis',(-0.211873077029416,-1.41064830464559E-17,0.97729719084324));
#26592=DIRECTION('center_axis',(-6.65798752924967E-17,1.,-1.71022579061586E-31));
#26593=DIRECTION('ref_axis',(-0.211873077029416,-1.41064830464559E-17,0.977297190843239));
#26594=DIRECTION('center_axis',(-6.65798752924967E-17,1.,-1.71022579061586E-31));
#26595=DIRECTION('ref_axis',(-0.211873077029416,-1.41064830464559E-17,0.97729719084324));
#26596=DIRECTION('center_axis',(-6.65798752924967E-17,1.,-1.71022579061586E-31));
#26597=DIRECTION('ref_axis',(-0.211873077029416,-1.41064830464559E-17,0.977297190843239));
#26598=DIRECTION('center_axis',(-6.65798752924967E-17,1.,-1.71022579061586E-31));
#26599=DIRECTION('ref_axis',(-0.211873077029416,-1.41064830464559E-17,0.97729719084324));
#26600=DIRECTION('center_axis',(-6.65798752924967E-17,1.,-1.71022579061586E-31));
#26601=DIRECTION('ref_axis',(-0.211873077029416,-1.41064830464559E-17,0.977297190843239));
#26602=DIRECTION('center_axis',(-6.65798752924967E-17,1.,-1.71022579061586E-31));
#26603=DIRECTION('ref_axis',(-0.211873077029416,-1.41064830464559E-17,0.97729719084324));
#26604=DIRECTION('center_axis',(-6.65798752924967E-17,1.,-1.71022579061586E-31));
#26605=DIRECTION('ref_axis',(-0.211873077029416,-1.41064830464559E-17,0.977297190843239));
#26606=DIRECTION('center_axis',(-6.65798752924967E-17,1.,-1.71022579061586E-31));
#26607=DIRECTION('ref_axis',(-0.211873077029416,-1.41064830464559E-17,0.97729719084324));
#26608=DIRECTION('center_axis',(-6.65798752924967E-17,1.,-1.71022579061586E-31));
#26609=DIRECTION('ref_axis',(-0.211873077029416,-1.41064830464559E-17,0.977297190843239));
#26610=DIRECTION('center_axis',(-6.65798752924967E-17,1.,-1.71022579061586E-31));
#26611=DIRECTION('ref_axis',(-0.211873077029416,-1.41064830464559E-17,0.97729719084324));
#26612=DIRECTION('center_axis',(-6.65798752924967E-17,1.,-1.71022579061586E-31));
#26613=DIRECTION('ref_axis',(-0.211873077029416,-1.41064830464559E-17,0.977297190843239));
#26614=DIRECTION('center_axis',(-6.65798752924967E-17,1.,-1.71022579061586E-31));
#26615=DIRECTION('ref_axis',(-0.211873077029416,-1.41064830464559E-17,0.97729719084324));
#26616=DIRECTION('center_axis',(-6.65798752924967E-17,1.,-1.71022579061586E-31));
#26617=DIRECTION('ref_axis',(-0.211873077029416,-1.41064830464559E-17,0.977297190843239));
#26618=DIRECTION('center_axis',(-6.65798752924967E-17,1.,-1.71022579061586E-31));
#26619=DIRECTION('ref_axis',(-0.211873077029416,-1.41064830464559E-17,0.97729719084324));
#26620=DIRECTION('center_axis',(-6.65798752924967E-17,1.,-1.71022579061586E-31));
#26621=DIRECTION('ref_axis',(-0.211873077029416,-1.41064830464559E-17,0.977297190843239));
#26622=DIRECTION('center_axis',(-6.65798752924967E-17,1.,-1.71022579061586E-31));
#26623=DIRECTION('ref_axis',(-0.211873077029416,-1.41064830464559E-17,0.97729719084324));
#26624=DIRECTION('center_axis',(-6.65798752924967E-17,1.,-1.71022579061586E-31));
#26625=DIRECTION('ref_axis',(-0.211873077029416,-1.41064830464559E-17,0.977297190843239));
#26626=DIRECTION('center_axis',(-6.65798752924967E-17,1.,-1.71022579061586E-31));
#26627=DIRECTION('ref_axis',(-0.211873077029416,-1.41064830464559E-17,0.97729719084324));
#26628=DIRECTION('center_axis',(-6.65798752924967E-17,1.,-1.71022579061586E-31));
#26629=DIRECTION('ref_axis',(-0.211873077029416,-1.41064830464559E-17,0.977297190843239));
#26630=DIRECTION('center_axis',(-6.65798752924967E-17,1.,-1.71022579061586E-31));
#26631=DIRECTION('ref_axis',(-0.211873077029416,-1.41064830464559E-17,0.97729719084324));
#26632=DIRECTION('center_axis',(-6.65798752924967E-17,1.,-1.71022579061586E-31));
#26633=DIRECTION('ref_axis',(-0.211873077029416,-1.41064830464559E-17,0.977297190843239));
#26634=DIRECTION('center_axis',(-6.65798752924967E-17,1.,-1.71022579061586E-31));
#26635=DIRECTION('ref_axis',(-0.211873077029416,-1.41064830464559E-17,0.97729719084324));
#26636=DIRECTION('center_axis',(-6.65798752924967E-17,1.,-1.71022579061586E-31));
#26637=DIRECTION('ref_axis',(-0.211873077029416,-1.41064830464559E-17,0.977297190843239));
#26638=DIRECTION('center_axis',(-6.65798752924967E-17,1.,-1.71022579061586E-31));
#26639=DIRECTION('ref_axis',(-0.211873077029416,-1.41064830464559E-17,0.97729719084324));
#26640=DIRECTION('center_axis',(-6.65798752924967E-17,1.,-1.71022579061586E-31));
#26641=DIRECTION('ref_axis',(-0.211873077029416,-1.41064830464559E-17,0.977297190843239));
#26642=DIRECTION('center_axis',(-6.65798752924967E-17,1.,-1.71022579061586E-31));
#26643=DIRECTION('ref_axis',(-0.211873077029416,-1.41064830464559E-17,0.97729719084324));
#26644=DIRECTION('center_axis',(-6.65798752924967E-17,1.,-1.71022579061586E-31));
#26645=DIRECTION('ref_axis',(-0.211873077029416,-1.41064830464559E-17,0.977297190843239));
#26646=DIRECTION('center_axis',(-6.65798752924967E-17,1.,-1.71022579061586E-31));
#26647=DIRECTION('ref_axis',(-0.211873077029416,-1.41064830464559E-17,0.97729719084324));
#26648=DIRECTION('center_axis',(-6.65798752924967E-17,1.,-1.71022579061586E-31));
#26649=DIRECTION('ref_axis',(-0.211873077029416,-1.41064830464559E-17,0.977297190843239));
#26650=DIRECTION('center_axis',(-6.65798752924967E-17,1.,-1.71022579061586E-31));
#26651=DIRECTION('ref_axis',(-0.211873077029416,-1.41064830464559E-17,0.97729719084324));
#26652=DIRECTION('center_axis',(-6.65798752924967E-17,1.,-1.71022579061586E-31));
#26653=DIRECTION('ref_axis',(-0.211873077029416,-1.41064830464559E-17,0.977297190843239));
#26654=DIRECTION('center_axis',(-6.65798752924967E-17,1.,-1.71022579061586E-31));
#26655=DIRECTION('ref_axis',(-0.211873077029416,-1.41064830464559E-17,0.97729719084324));
#26656=DIRECTION('center_axis',(-6.65798752924967E-17,1.,-1.71022579061586E-31));
#26657=DIRECTION('ref_axis',(-0.211873077029416,-1.41064830464559E-17,0.977297190843239));
#26658=DIRECTION('center_axis',(-6.65798752924967E-17,1.,-1.71022579061586E-31));
#26659=DIRECTION('ref_axis',(-0.211873077029416,-1.41064830464559E-17,0.97729719084324));
#26660=DIRECTION('center_axis',(-6.65798752924967E-17,1.,-1.71022579061586E-31));
#26661=DIRECTION('ref_axis',(-0.211873077029416,-1.41064830464559E-17,0.977297190843239));
#26662=DIRECTION('center_axis',(-6.65798752924967E-17,1.,-1.71022579061586E-31));
#26663=DIRECTION('ref_axis',(-0.211873077029416,-1.41064830464559E-17,0.97729719084324));
#26664=DIRECTION('center_axis',(-6.65798752924967E-17,1.,-1.71022579061586E-31));
#26665=DIRECTION('ref_axis',(-0.211873077029416,-1.41064830464559E-17,0.977297190843239));
#26666=DIRECTION('center_axis',(-6.65798752924967E-17,1.,-1.71022579061586E-31));
#26667=DIRECTION('ref_axis',(-0.211873077029416,-1.41064830464559E-17,0.97729719084324));
#26668=DIRECTION('center_axis',(-6.65798752924967E-17,1.,-1.71022579061586E-31));
#26669=DIRECTION('ref_axis',(-0.211873077029416,-1.41064830464559E-17,0.977297190843239));
#26670=DIRECTION('center_axis',(-6.65798752924967E-17,1.,-1.71022579061586E-31));
#26671=DIRECTION('ref_axis',(-0.211873077029416,-1.41064830464559E-17,0.97729719084324));
#26672=DIRECTION('center_axis',(-6.65798752924967E-17,1.,-1.71022579061586E-31));
#26673=DIRECTION('ref_axis',(-0.211873077029416,-1.41064830464559E-17,0.977297190843239));
#26674=DIRECTION('center_axis',(-6.65798752924967E-17,1.,-1.71022579061586E-31));
#26675=DIRECTION('ref_axis',(-0.211873077029416,-1.41064830464559E-17,0.97729719084324));
#26676=DIRECTION('center_axis',(-6.65798752924967E-17,1.,-1.71022579061586E-31));
#26677=DIRECTION('ref_axis',(-0.211873077029416,-1.41064830464559E-17,0.977297190843239));
#26678=DIRECTION('center_axis',(-6.65798752924967E-17,1.,-1.71022579061586E-31));
#26679=DIRECTION('ref_axis',(-0.211873077029416,-1.41064830464559E-17,0.97729719084324));
#26680=DIRECTION('center_axis',(-6.65798752924967E-17,1.,-1.71022579061586E-31));
#26681=DIRECTION('ref_axis',(-0.211873077029416,-1.41064830464559E-17,0.977297190843239));
#26682=DIRECTION('center_axis',(-6.65798752924967E-17,1.,-1.71022579061586E-31));
#26683=DIRECTION('ref_axis',(-0.211873077029416,-1.41064830464559E-17,0.97729719084324));
#26684=DIRECTION('center_axis',(-6.65798752924967E-17,1.,-1.71022579061586E-31));
#26685=DIRECTION('ref_axis',(-0.211873077029416,-1.41064830464559E-17,0.977297190843239));
#26686=DIRECTION('center_axis',(-6.65798752924967E-17,1.,-1.71022579061586E-31));
#26687=DIRECTION('ref_axis',(-0.211873077029416,-1.41064830464559E-17,0.97729719084324));
#26688=DIRECTION('center_axis',(-6.65798752924967E-17,1.,-1.71022579061586E-31));
#26689=DIRECTION('ref_axis',(-0.211873077029416,-1.41064830464559E-17,0.977297190843239));
#26690=DIRECTION('center_axis',(-6.65798752924967E-17,1.,-1.71022579061586E-31));
#26691=DIRECTION('ref_axis',(-0.211873077029416,-1.41064830464559E-17,0.97729719084324));
#26692=DIRECTION('center_axis',(-6.65798752924967E-17,1.,-1.71022579061586E-31));
#26693=DIRECTION('ref_axis',(-0.211873077029416,-1.41064830464559E-17,0.977297190843239));
#26694=DIRECTION('center_axis',(-6.65798752924967E-17,1.,-1.71022579061586E-31));
#26695=DIRECTION('ref_axis',(-0.211873077029416,-1.41064830464559E-17,0.97729719084324));
#26696=DIRECTION('center_axis',(-6.65798752924967E-17,1.,-1.71022579061586E-31));
#26697=DIRECTION('ref_axis',(-0.211873077029416,-1.41064830464559E-17,0.977297190843239));
#26698=DIRECTION('center_axis',(-6.65798752924967E-17,1.,-1.71022579061586E-31));
#26699=DIRECTION('ref_axis',(-0.211873077029416,-1.41064830464559E-17,0.97729719084324));
#26700=DIRECTION('center_axis',(-6.65798752924967E-17,1.,-1.71022579061586E-31));
#26701=DIRECTION('ref_axis',(-0.211873077029416,-1.41064830464559E-17,0.977297190843239));
#26702=DIRECTION('center_axis',(-6.65798752924967E-17,1.,-1.71022579061586E-31));
#26703=DIRECTION('ref_axis',(-0.211873077029416,-1.41064830464559E-17,0.97729719084324));
#26704=DIRECTION('center_axis',(-6.65798752924967E-17,1.,-1.71022579061586E-31));
#26705=DIRECTION('ref_axis',(-0.211873077029416,-1.41064830464559E-17,0.977297190843239));
#26706=DIRECTION('center_axis',(-6.65798752924967E-17,1.,-1.71022579061586E-31));
#26707=DIRECTION('ref_axis',(-0.211873077029416,-1.41064830464559E-17,0.97729719084324));
#26708=DIRECTION('center_axis',(-6.65798752924967E-17,1.,-1.71022579061586E-31));
#26709=DIRECTION('ref_axis',(-0.211873077029416,-1.41064830464559E-17,0.977297190843239));
#26710=DIRECTION('center_axis',(-6.65798752924967E-17,1.,-1.71022579061586E-31));
#26711=DIRECTION('ref_axis',(-0.211873077029416,-1.41064830464559E-17,0.97729719084324));
#26712=DIRECTION('center_axis',(-6.65798752924967E-17,1.,-1.71022579061586E-31));
#26713=DIRECTION('ref_axis',(-0.211873077029416,-1.41064830464559E-17,0.977297190843239));
#26714=DIRECTION('center_axis',(-6.65798752924967E-17,1.,-1.71022579061586E-31));
#26715=DIRECTION('ref_axis',(-0.211873077029416,-1.41064830464559E-17,0.97729719084324));
#26716=DIRECTION('center_axis',(-6.65798752924967E-17,1.,-1.71022579061586E-31));
#26717=DIRECTION('ref_axis',(-0.211873077029416,-1.41064830464559E-17,0.977297190843239));
#26718=DIRECTION('center_axis',(-6.65798752924967E-17,1.,-1.71022579061586E-31));
#26719=DIRECTION('ref_axis',(-0.211873077029416,-1.41064830464559E-17,0.97729719084324));
#26720=DIRECTION('center_axis',(-6.65798752924967E-17,1.,-1.71022579061586E-31));
#26721=DIRECTION('ref_axis',(-0.211873077029416,-1.41064830464559E-17,0.977297190843239));
#26722=DIRECTION('center_axis',(-6.65798752924967E-17,1.,-1.71022579061586E-31));
#26723=DIRECTION('ref_axis',(-0.211873077029416,-1.41064830464559E-17,0.97729719084324));
#26724=DIRECTION('center_axis',(-6.65798752924967E-17,1.,-1.71022579061586E-31));
#26725=DIRECTION('ref_axis',(-0.211873077029416,-1.41064830464559E-17,0.977297190843239));
#26726=DIRECTION('center_axis',(-6.65798752924967E-17,1.,-1.71022579061586E-31));
#26727=DIRECTION('ref_axis',(-0.211873077029416,-1.41064830464559E-17,0.97729719084324));
#26728=DIRECTION('center_axis',(-6.65798752924967E-17,1.,-1.71022579061586E-31));
#26729=DIRECTION('ref_axis',(-0.211873077029416,-1.41064830464559E-17,0.977297190843239));
#26730=DIRECTION('center_axis',(-6.65798752924967E-17,1.,-1.71022579061586E-31));
#26731=DIRECTION('ref_axis',(-0.211873077029416,-1.41064830464559E-17,0.97729719084324));
#26732=DIRECTION('center_axis',(6.65798752924967E-17,-1.,1.71022579061586E-31));
#26733=DIRECTION('ref_axis',(-0.211873077029416,-1.41064830464559E-17,0.977297190843239));
#26734=DIRECTION('center_axis',(-6.65798752924967E-17,1.,-1.71022579061586E-31));
#26735=DIRECTION('ref_axis',(-0.211873077029416,-1.41064830464559E-17,0.977297190843239));
#26736=DIRECTION('center_axis',(-6.65798752924967E-17,1.,-1.71022579061586E-31));
#26737=DIRECTION('ref_axis',(-0.211873077029416,-1.41064830464559E-17,0.97729719084324));
#26738=DIRECTION('center_axis',(-6.65798752924967E-17,1.,-1.71022579061586E-31));
#26739=DIRECTION('ref_axis',(-0.211873077029416,-1.41064830464559E-17,0.97729719084324));
#26740=DIRECTION('center_axis',(6.65798752924967E-17,-1.,1.71022579061586E-31));
#26741=DIRECTION('ref_axis',(0.211873077029416,1.41064830464559E-17,-0.977297190843239));
#26742=DIRECTION('center_axis',(-6.65798752924967E-17,1.,-1.71022579061586E-31));
#26743=DIRECTION('ref_axis',(-0.211873077029416,-1.41064830464559E-17,0.977297190843239));
#26744=DIRECTION('center_axis',(-6.65798752924967E-17,1.,-1.71022579061586E-31));
#26745=DIRECTION('ref_axis',(0.211873077029416,1.41064830464559E-17,-0.97729719084324));
#26746=DIRECTION('',(-6.65798752924967E-17,1.,-1.71022579061586E-31));
#32380=CARTESIAN_POINT('',(0.,0.,0.));
#32381=CARTESIAN_POINT('Origin',(0.0121040592752336,-0.01,0.00446113764208535));
#32382=CARTESIAN_POINT('',(0.0122678470666214,-0.01,0.00398872515347788));
#32383=CARTESIAN_POINT('',(0.0122678470666214,-0.0155,0.00398872515347788));
#32384=CARTESIAN_POINT('',(0.0122678470666291,-0.01000000000001,0.00398872515348977));
#32385=CARTESIAN_POINT('',(0.0119220873914306,-0.01,0.0049268481031072));
#32386=CARTESIAN_POINT('Origin',(0.0121040592752413,-0.01000000000001,0.00446113764209724));
#32387=CARTESIAN_POINT('',(0.0119220873914306,-0.0155,0.0049268481031072));
#32388=CARTESIAN_POINT('',(0.0119220873914382,-0.01000000000001,0.00492684810311909));
#32389=CARTESIAN_POINT('Origin',(0.0121040592752413,-0.01550000000001,0.00446113764209724));
#32390=CARTESIAN_POINT('Origin',(0.0113653930429603,-0.01,0.00610228162075688));
#32391=CARTESIAN_POINT('',(0.0115933339737932,-0.01,0.00565726147284101));
#32392=CARTESIAN_POINT('',(0.0115933339737932,-0.0155,0.00565726147284101));
#32393=CARTESIAN_POINT('',(0.0115933339738008,-0.01000000000001,0.0056572614728529));
#32394=CARTESIAN_POINT('',(0.0111203777280115,-0.01,0.00653813422822932));
#32395=CARTESIAN_POINT('Origin',(0.011365393042968,-0.01000000000001,0.00610228162076877));
#32396=CARTESIAN_POINT('',(0.0111203777280115,-0.0155,0.00653813422822932));
#32397=CARTESIAN_POINT('',(0.0111203777280192,-0.01000000000001,0.00653813422824121));
#32398=CARTESIAN_POINT('Origin',(0.011365393042968,-0.01550000000001,0.00610228162076877));
#32399=CARTESIAN_POINT('Origin',(0.0104055123630489,-0.01,0.00762465162892286));
#32400=CARTESIAN_POINT('',(0.0106931698223871,-0.01,0.00721568563267485));
#32401=CARTESIAN_POINT('',(0.0106931698223871,-0.0155,0.00721568563267485));
#32402=CARTESIAN_POINT('',(0.0106931698223947,-0.01000000000001,0.00721568563268675));
#32403=CARTESIAN_POINT('',(0.010102222561359,-0.01,0.00802216300761643));
#32404=CARTESIAN_POINT('Origin',(0.0104055123630566,-0.01000000000001,0.00762465162893475));
#32405=CARTESIAN_POINT('',(0.010102222561359,-0.0155,0.00802216300761643));
#32406=CARTESIAN_POINT('',(0.0101022225613666,-0.01000000000001,0.00802216300762832));
#32407=CARTESIAN_POINT('Origin',(0.0104055123630566,-0.01550000000001,0.00762465162893475));
#32408=CARTESIAN_POINT('Origin',(0.00924310022108555,-0.01,0.00899861646604452));
#32409=CARTESIAN_POINT('',(0.00958487528368847,-0.01,0.00863366467938941));
#32410=CARTESIAN_POINT('',(0.00958487528368847,-0.0155,0.00863366467938941));
#32411=CARTESIAN_POINT('',(0.00958487528369612,-0.01000000000001,0.00863366467940131));
#32412=CARTESIAN_POINT('',(0.00888743912365737,-0.01,0.00935004950913547));
#32413=CARTESIAN_POINT('Origin',(0.00924310022109321,-0.01000000000001,
0.00899861646605642));
#32414=CARTESIAN_POINT('',(0.00888743912365737,-0.0155,0.00935004950913547));
#32415=CARTESIAN_POINT('',(0.00888743912366502,-0.01000000000001,0.00935004950914736));
#32416=CARTESIAN_POINT('Origin',(0.00924310022109321,-0.01550000000001,
0.00899861646605642));
#32417=CARTESIAN_POINT('Origin',(0.00790078164718944,-0.01,0.0101974334694291));
#32418=CARTESIAN_POINT('',(0.00829002205022697,-0.01,0.00988359926376768));
#32419=CARTESIAN_POINT('',(0.00829002205022697,-0.0155,0.00988359926376768));
#32420=CARTESIAN_POINT('',(0.00829002205023463,-0.01000000000001,0.00988359926377957));
#32421=CARTESIAN_POINT('',(0.0074996717927259,-0.01,0.0104959479324828));
#32422=CARTESIAN_POINT('Origin',(0.0079007816471971,-0.01000000000001,0.010197433469441));
#32423=CARTESIAN_POINT('',(0.0074996717927259,-0.0155,0.0104959479324828));
#32424=CARTESIAN_POINT('',(0.00749967179273355,-0.01000000000001,0.0104959479324947));
#32425=CARTESIAN_POINT('Origin',(0.0079007816471971,-0.01550000000001,0.010197433469441));
#32426=CARTESIAN_POINT('Origin',(0.00640468334553672,-0.01,0.01119776902974));
#32427=CARTESIAN_POINT('',(0.00683381296731816,-0.01,0.0109411608309043));
#32428=CARTESIAN_POINT('',(0.00683381296731816,-0.0155,0.0109411608309043));
#32429=CARTESIAN_POINT('',(0.00683381296732582,-0.01000000000001,0.0109411608309161));
#32430=CARTESIAN_POINT('',(0.00596593188109928,-0.01,0.0114375546682883));
#32431=CARTESIAN_POINT('Origin',(0.00640468334554438,-0.01000000000001,
0.0111977690297519));
#32432=CARTESIAN_POINT('',(0.00596593188109928,-0.0155,0.0114375546682883));
#32433=CARTESIAN_POINT('',(0.00596593188110694,-0.01000000000001,0.0114375546683002));
#32434=CARTESIAN_POINT('Origin',(0.00640468334554438,-0.01550000000001,
0.0111977690297519));
#32435=CARTESIAN_POINT('Origin',(0.00478392516778247,-0.01,0.0119801527531604));
#32436=CARTESIAN_POINT('',(0.0052445914883475,-0.01,0.0117857651478533));
#32437=CARTESIAN_POINT('',(0.0052445914883475,-0.0155,0.0117857651478533));
#32438=CARTESIAN_POINT('',(0.00524459148835515,-0.01000000000001,0.0117857651478652));
#32439=CARTESIAN_POINT('',(0.004316071891554,-0.01,0.0121565424125011));
#32440=CARTESIAN_POINT('Origin',(0.00478392516779012,-0.01000000000001,
0.0119801527531723));
#32441=CARTESIAN_POINT('',(0.004316071891554,-0.0155,0.0121565424125011));
#32442=CARTESIAN_POINT('',(0.00431607189156165,-0.01000000000001,0.012156542412513));
#32443=CARTESIAN_POINT('Origin',(0.00478392516779012,-0.01550000000001,
0.0119801527531723));
#32444=CARTESIAN_POINT('Origin',(0.00307005332827152,-0.01,0.0125293564304624));
#32445=CARTESIAN_POINT('',(0.00355329000169056,-0.01,0.0124009729523085));
#32446=CARTESIAN_POINT('',(0.00355329000169056,-0.0155,0.0124009729523085));
#32447=CARTESIAN_POINT('',(0.00355329000169822,-0.01000000000001,0.0124009729523203));
#32448=CARTESIAN_POINT('',(0.00258220447209863,-0.01,0.0126389168865166));
#32449=CARTESIAN_POINT('Origin',(0.00307005332827917,-0.01000000000001,
0.0125293564304743));
#32450=CARTESIAN_POINT('',(0.00258220447209862,-0.0155,0.0126389168865166));
#32451=CARTESIAN_POINT('',(0.00258220447210627,-0.01000000000001,0.0126389168865285));
#32452=CARTESIAN_POINT('Origin',(0.00307005332827917,-0.01550000000001,
0.0125293564304743));
#32453=CARTESIAN_POINT('Origin',(0.00129642639285968,-0.01,0.0128346904367771));
#32454=CARTESIAN_POINT('',(0.00179282776695818,-0.01,0.0127748099241446));
#32455=CARTESIAN_POINT('',(0.00179282776695818,-0.0155,0.0127748099241446));
#32456=CARTESIAN_POINT('',(0.00179282776696584,-0.01000000000001,0.0127748099241565));
#32457=CARTESIAN_POINT('',(0.000798077379807918,-0.01,0.0128752892198909));
#32458=CARTESIAN_POINT('Origin',(0.00129642639286733,-0.01000000000001,
0.012834690436789));
#32459=CARTESIAN_POINT('',(0.000798077379807918,-0.0155,0.0128752892198909));
#32460=CARTESIAN_POINT('',(0.000798077379815572,-0.01000000000001,0.0128752892199028));
#32461=CARTESIAN_POINT('Origin',(0.00129642639286733,-0.01550000000001,
0.012834690436789));
#32462=CARTESIAN_POINT('Origin',(-0.000502434007626007,-0.01,0.0128902117929839));
#32463=CARTESIAN_POINT('',(-2.52982094668758E-6,-0.01,0.0128999997519382));
#32464=CARTESIAN_POINT('',(-2.52982094668715E-6,-0.0155,0.0128999997519382));
#32465=CARTESIAN_POINT('',(-2.52982093903355E-6,-0.01000000000001,0.0128999997519501));
#32466=CARTESIAN_POINT('',(-0.00100158338088122,-0.01,0.0128610586940245));
#32467=CARTESIAN_POINT('Origin',(-0.000502434007618353,-0.01000000000001,
0.0128902117929958));
#32468=CARTESIAN_POINT('',(-0.00100158338088122,-0.0155,0.0128610586940245));
#32469=CARTESIAN_POINT('',(-0.00100158338087356,-0.01000000000001,0.0128610586940364));
#32470=CARTESIAN_POINT('Origin',(-0.000502434007618352,-0.01550000000001,
0.0128902117929958));
#32471=CARTESIAN_POINT('Origin',(-0.00229151510166345,-0.01,0.0126948398390388));
#32472=CARTESIAN_POINT('',(-0.00179783816876445,-0.01,0.0127741057580926));
#32473=CARTESIAN_POINT('',(-0.00179783816876445,-0.0155,0.0127741057580926));
#32474=CARTESIAN_POINT('',(-0.0017978381687568,-0.01000000000001,0.0127741057581045));
#32475=CARTESIAN_POINT('',(-0.00278174946034568,-0.01,0.0125965022899163));
#32476=CARTESIAN_POINT('Origin',(-0.00229151510165579,-0.01000000000001,
0.0126948398390507));
#32477=CARTESIAN_POINT('',(-0.00278174946034568,-0.0155,0.0125965022899163));
#32478=CARTESIAN_POINT('',(-0.00278174946035758,-0.01000000000001,0.012596502289924));
#32479=CARTESIAN_POINT('Origin',(-0.00229151510165579,-0.01550000000001,
0.0126948398390507));
#32480=CARTESIAN_POINT('Origin',(-0.00403599446080683,-0.01,0.0122523772677932));
#32481=CARTESIAN_POINT('',(-0.00355815364163782,-0.01,0.0123995783259956));
#32482=CARTESIAN_POINT('',(-0.00355815364163782,-0.0155,0.0123995783259956));
#32483=CARTESIAN_POINT('',(-0.00355815364164971,-0.01000000000001,0.0123995783260032));
#32484=CARTESIAN_POINT('',(-0.00450777195075764,-0.01,0.0120867692970439));
#32485=CARTESIAN_POINT('Origin',(-0.00403599446081873,-0.01000000000001,
0.0122523772678009));
#32486=CARTESIAN_POINT('',(-0.00450777195075764,-0.0155,0.0120867692970439));
#32487=CARTESIAN_POINT('',(-0.00450777195076953,-0.01000000000001,0.0120867692970515));
#32488=CARTESIAN_POINT('Origin',(-0.00403599446081873,-0.01550000000001,
0.0122523772678009));
#32489=CARTESIAN_POINT('Origin',(-0.00570191777864627,-0.01,0.0115714361099027));
#32490=CARTESIAN_POINT('',(-0.0052492137012165,-0.01,0.0117837072060944));
#32491=CARTESIAN_POINT('',(-0.0052492137012165,-0.0155,0.0117837072060944));
#32492=CARTESIAN_POINT('',(-0.00524921370122839,-0.01000000000001,0.0117837072061021));
#32493=CARTESIAN_POINT('',(-0.0061460557876627,-0.01,0.0113417810883008));
#32494=CARTESIAN_POINT('Origin',(-0.00570191777865816,-0.01000000000001,
0.0115714361099103));
#32495=CARTESIAN_POINT('',(-0.0061460557876627,-0.0155,0.0113417810883008));
#32496=CARTESIAN_POINT('',(-0.00614605578767459,-0.01000000000001,0.0113417810883085));
#32497=CARTESIAN_POINT('Origin',(-0.00570191777865816,-0.01550000000001,
0.0115714361099103));
#32498=CARTESIAN_POINT('Origin',(-0.0072568597527597,-0.01,0.0106652701104462));
#32499=CARTESIAN_POINT('',(-0.0068381037869931,-0.01,0.0109384796291949));
#32500=CARTESIAN_POINT('',(-0.0068381037869931,-0.0155,0.0109384796291949));
#32501=CARTESIAN_POINT('',(-0.00683810378700499,-0.01000000000001,0.0109384796292026));
#32502=CARTESIAN_POINT('',(-0.00766471363969576,-0.01,0.0103760380117588));
#32503=CARTESIAN_POINT('Origin',(-0.00725685975277159,-0.01000000000001,
0.0106652701104539));
#32504=CARTESIAN_POINT('',(-0.00766471363969575,-0.0155,0.0103760380117588));
#32505=CARTESIAN_POINT('',(-0.00766471363970765,-0.01000000000001,0.0103760380117664));
#32506=CARTESIAN_POINT('Origin',(-0.00725685975277159,-0.01550000000001,
0.0106652701104539));
#32507=CARTESIAN_POINT('Origin',(-0.00867055520634127,-0.01,0.00955151675985495));
#32508=CARTESIAN_POINT('',(-0.00829389796078364,-0.01,0.00988034698864926));
#32509=CARTESIAN_POINT('',(-0.00829389796078364,-0.0155,0.00988034698864926));
#32510=CARTESIAN_POINT('',(-0.00829389796079552,-0.01000000000001,0.00988034698865692));
#32511=CARTESIAN_POINT('',(-0.00903418655921466,-0.01,0.00920833715788611));
#32512=CARTESIAN_POINT('Origin',(-0.00867055520635317,-0.01000000000001,
0.0095515167598626));
#32513=CARTESIAN_POINT('',(-0.00903418655921466,-0.0155,0.00920833715788611));
#32514=CARTESIAN_POINT('',(-0.00903418655922655,-0.01000000000001,0.00920833715789376));
#32515=CARTESIAN_POINT('Origin',(-0.00867055520635317,-0.01550000000001,
0.0095515167598626));
#32516=CARTESIAN_POINT('Origin',(-0.00991548816544177,-0.01,0.0082518540002223));
#32517=CARTESIAN_POINT('',(-0.00958826084493661,-0.01,0.0086299046326977));
#32518=CARTESIAN_POINT('',(-0.00958826084493661,-0.0155,0.0086299046326977));
#32519=CARTESIAN_POINT('',(-0.0095882608449485,-0.01000000000001,0.00862990463270536));
#32520=CARTESIAN_POINT('',(-0.0102278193135934,-0.01,0.00786140649556347));
#32521=CARTESIAN_POINT('Origin',(-0.00991548816545366,-0.01000000000001,
0.00825185400022996));
#32522=CARTESIAN_POINT('',(-0.0102278193135934,-0.0155,0.00786140649556347));
#32523=CARTESIAN_POINT('',(-0.0102278193136052,-0.01000000000001,0.00786140649557113));
#32524=CARTESIAN_POINT('Origin',(-0.00991548816545366,-0.01550000000001,
0.00825185400022996));
#32525=CARTESIAN_POINT('Origin',(-0.0109674274261026,-0.01,0.0067915782888202));
#32526=CARTESIAN_POINT('',(-0.010695999138228,-0.01,0.00721149099944164));
#32527=CARTESIAN_POINT('',(-0.010695999138228,-0.0155,0.00721149099944164));
#32528=CARTESIAN_POINT('',(-0.0106959991382398,-0.01000000000001,0.0072114909994493));
#32529=CARTESIAN_POINT('',(-0.011222379199005,-0.01,0.00636146249802205));
#32530=CARTESIAN_POINT('Origin',(-0.0109674274261145,-0.01000000000001,
0.00679157828882786));
#32531=CARTESIAN_POINT('',(-0.011222379199005,-0.0155,0.00636146249802205));
#32532=CARTESIAN_POINT('',(-0.0112223791990169,-0.01000000000001,0.00636146249802971));
#32533=CARTESIAN_POINT('Origin',(-0.0109674274261145,-0.01550000000001,
0.00679157828882786));
#32534=CARTESIAN_POINT('Origin',(-0.0118058981871781,-0.01,0.005199112231332));
#32535=CARTESIAN_POINT('',(-0.0115955519748124,-0.01,0.00565271389683093));
#32536=CARTESIAN_POINT('',(-0.0115955519748124,-0.0155,0.00565271389683093));
#32537=CARTESIAN_POINT('',(-0.0115955519748243,-0.01000000000001,0.00565271389683857));
#32538=CARTESIAN_POINT('',(-0.0119985082385752,-0.01,0.00473769986901296));
#32539=CARTESIAN_POINT('Origin',(-0.01180589818719,-0.01000000000001,0.00519911223133965));
#32540=CARTESIAN_POINT('',(-0.0119985082385752,-0.0155,0.00473769986901296));
#32541=CARTESIAN_POINT('',(-0.0119985082385871,-0.01000000000001,0.00473769986902062));
#32542=CARTESIAN_POINT('Origin',(-0.01180589818719,-0.01550000000001,0.00519911223133965));
#32543=CARTESIAN_POINT('Origin',(-0.0124145805690504,-0.01,0.00350545136816342));
#32544=CARTESIAN_POINT('',(-0.012269410581952,-0.01,0.00398391314808515));
#32545=CARTESIAN_POINT('',(-0.012269410581952,-0.0155,0.00398391314808515));
#32546=CARTESIAN_POINT('',(-0.0122694105819639,-0.01000000000001,0.00398391314809281));
#32547=CARTESIAN_POINT('',(-0.0125410999633822,-0.01,0.00302172330110727));
#32548=CARTESIAN_POINT('Origin',(-0.0124145805690623,-0.01000000000001,
0.00350545136817107));
#32549=CARTESIAN_POINT('',(-0.0125410999633822,-0.0155,0.00302172330110727));
#32550=CARTESIAN_POINT('',(-0.0125410999633941,-0.01000000000001,0.00302172330111493));
#32551=CARTESIAN_POINT('Origin',(-0.0124145805690623,-0.01550000000001,
0.00350545136817107));
#32552=CARTESIAN_POINT('Origin',(-0.0127816272615221,-0.01,0.0017435608815054));
#32553=CARTESIAN_POINT('',(-0.0127044590683616,-0.01,0.00223757006154593));
#32554=CARTESIAN_POINT('',(-0.0127044590683616,-0.0155,0.00223757006154593));
#32555=CARTESIAN_POINT('',(-0.0127044590683735,-0.01000000000001,0.00223757006155359));
#32556=CARTESIAN_POINT('',(-0.0128395934426919,-0.01,0.00124693232630483));
#32557=CARTESIAN_POINT('Origin',(-0.012781627261534,-0.01000000000001,0.00174356088151305));
#32558=CARTESIAN_POINT('',(-0.0128395934426919,-0.0155,0.00124693232630483));
#32559=CARTESIAN_POINT('',(-0.0128395934427038,-0.01000000000001,0.00124693232631249));
#32560=CARTESIAN_POINT('Origin',(-0.012781627261534,-0.01550000000001,0.00174356088151305));
#32561=CARTESIAN_POINT('Origin',(-0.0128998941182339,-0.01,-5.22660344400411E-5));
#32562=CARTESIAN_POINT('',(-0.0128922297101135,-0.01,0.00044767521895696));
#32563=CARTESIAN_POINT('',(-0.0128922297101135,-0.0155,0.00044767521895696));
#32564=CARTESIAN_POINT('',(-0.0128922297101254,-0.01000000000001,0.000447675218964614));
#32565=CARTESIAN_POINT('',(-0.0128881788404607,-0.01,-0.000552128767864633));
#32566=CARTESIAN_POINT('Origin',(-0.0128998941182458,-0.01000000000001,
-5.22660344323867E-5));
#32567=CARTESIAN_POINT('',(-0.0128881788404607,-0.0155,-0.000552128767864633));
#32568=CARTESIAN_POINT('',(-0.0128881788404726,-0.01000000000001,-0.000552128767856978));
#32569=CARTESIAN_POINT('Origin',(-0.0128998941182458,-0.01550000000001,
-5.22660344323867E-5));
#32570=CARTESIAN_POINT('Origin',(-0.0127670792093463,-0.01,-0.00184707565147683));
#32571=CARTESIAN_POINT('',(-0.012829067765252,-0.01,-0.001350933112546));
#32572=CARTESIAN_POINT('',(-0.012829067765252,-0.0155,-0.001350933112546));
#32573=CARTESIAN_POINT('',(-0.0128290677652638,-0.01000000000001,-0.00135093311253835));
#32574=CARTESIAN_POINT('',(-0.012685910497186,-0.01,-0.00234044330360477));
#32575=CARTESIAN_POINT('Origin',(-0.0127670792093582,-0.01000000000001,
-0.00184707565146918));
#32576=CARTESIAN_POINT('',(-0.012685910497186,-0.0155,-0.00234044330360477));
#32577=CARTESIAN_POINT('',(-0.0126859104971979,-0.01000000000001,-0.00234044330359712));
#32578=CARTESIAN_POINT('Origin',(-0.0127670792093582,-0.01550000000001,
-0.00184707565146918));
#32579=CARTESIAN_POINT('Origin',(-0.0123857676259861,-0.01,-0.00360593404197504));
#32580=CARTESIAN_POINT('',(-0.0125162026091882,-0.01,-0.00312324706767692));
#32581=CARTESIAN_POINT('',(-0.0125162026091882,-0.0155,-0.00312324706767692));
#32582=CARTESIAN_POINT('',(-0.0125162026091958,-0.01000000000001,-0.00312324706768881));
#32583=CARTESIAN_POINT('',(-0.0122367253360928,-0.01,-0.00408320377265504));
#32584=CARTESIAN_POINT('Origin',(-0.0123857676259938,-0.01000000000001,
-0.00360593404198693));
#32585=CARTESIAN_POINT('',(-0.0122367253360928,-0.0155,-0.00408320377265504));
#32586=CARTESIAN_POINT('',(-0.0122367253361005,-0.01000000000001,-0.00408320377266693));
#32587=CARTESIAN_POINT('Origin',(-0.0123857676259938,-0.01550000000001,
-0.00360593404198693));
#32588=CARTESIAN_POINT('Origin',(-0.011763381164388,-0.01,-0.00529460702803539));
#32589=CARTESIAN_POINT('',(-0.011959723806306,-0.01,-0.00483477057127637));
#32590=CARTESIAN_POINT('',(-0.011959723806306,-0.0155,-0.00483477057127637));
#32591=CARTESIAN_POINT('',(-0.0119597238063136,-0.01000000000001,-0.00483477057128826));
#32592=CARTESIAN_POINT('',(-0.0115493662354015,-0.01,-0.00574648932484605));
#32593=CARTESIAN_POINT('Origin',(-0.0117633811643957,-0.01000000000001,
-0.00529460702804728));
#32594=CARTESIAN_POINT('',(-0.0115493662354015,-0.0155,-0.00574648932484605));
#32595=CARTESIAN_POINT('',(-0.0115493662354091,-0.01000000000001,-0.00574648932485794));
#32596=CARTESIAN_POINT('Origin',(-0.0117633811643957,-0.01550000000001,
-0.00529460702804728));
#32597=CARTESIAN_POINT('Origin',(-0.0109120338690729,-0.01,-0.00688022651082125));
#32598=CARTESIAN_POINT('',(-0.0111704625835182,-0.01,-0.00645219076517593));
#32599=CARTESIAN_POINT('',(-0.0111704625835182,-0.0155,-0.00645219076517593));
#32600=CARTESIAN_POINT('',(-0.0111704625835258,-0.01000000000001,-0.00645219076518782));
#32601=CARTESIAN_POINT('',(-0.0106372118581474,-0.01,-0.00729792599886364));
#32602=CARTESIAN_POINT('Origin',(-0.0109120338690805,-0.01000000000001,
-0.00688022651083314));
#32603=CARTESIAN_POINT('',(-0.0106372118581474,-0.0155,-0.00729792599886364));
#32604=CARTESIAN_POINT('',(-0.010637211858155,-0.01000000000001,-0.00729792599887552));
#32605=CARTESIAN_POINT('Origin',(-0.0109120338690805,-0.01550000000001,
-0.00688022651083314));
#32606=CARTESIAN_POINT('Origin',(-0.0098482962467508,-0.01,-0.00833193021071565));
#32607=CARTESIAN_POINT('',(-0.0101637810127551,-0.01,-0.00794402640508956));
#32608=CARTESIAN_POINT('',(-0.0101637810127551,-0.0155,-0.00794402640508956));
#32609=CARTESIAN_POINT('',(-0.0101637810127627,-0.01000000000001,-0.00794402640510145));
#32610=CARTESIAN_POINT('',(-0.0095180162517236,-0.01,-0.00870731684458113));
#32611=CARTESIAN_POINT('Origin',(-0.00984829624675845,-0.01000000000001,
-0.00833193021072754));
#32612=CARTESIAN_POINT('',(-0.0095180162517236,-0.0155,-0.00870731684458113));
#32613=CARTESIAN_POINT('',(-0.00951801625173126,-0.01000000000001,-0.00870731684459302));
#32614=CARTESIAN_POINT('Origin',(-0.00984829624675845,-0.01550000000001,
-0.00833193021072754));
#32615=CARTESIAN_POINT('Origin',(-0.00859287274025656,-0.01,-0.00962146236648858));
#32616=CARTESIAN_POINT('',(-0.0089592730057083,-0.01,-0.00928124060722424));
#32617=CARTESIAN_POINT('',(-0.0089592730057083,-0.0155,-0.00928124060722424));
#32618=CARTESIAN_POINT('',(-0.00895927300571595,-0.01000000000001,-0.00928124060723613));
#32619=CARTESIAN_POINT('',(-0.00821356328554307,-0.01,-0.00994722967234497));
#32620=CARTESIAN_POINT('Origin',(-0.00859287274026421,-0.01000000000001,
-0.00962146236650047));
#32621=CARTESIAN_POINT('',(-0.00821356328554307,-0.0155,-0.00994722967234497));
#32622=CARTESIAN_POINT('',(-0.00821356328555072,-0.01000000000001,-0.00994722967235687));
#32623=CARTESIAN_POINT('Origin',(-0.00859287274026421,-0.01550000000001,
-0.00962146236650047));
#32624=CARTESIAN_POINT('Origin',(-0.00717019874012118,-0.01,-0.0107237237015491));
#32625=CARTESIAN_POINT('',(-0.00758038294062734,-0.01,-0.010437806018194));
#32626=CARTESIAN_POINT('',(-0.00758038294062734,-0.0155,-0.010437806018194));
#32627=CARTESIAN_POINT('',(-0.00758038294063499,-0.01000000000001,-0.0104378060182059));
#32628=CARTESIAN_POINT('',(-0.00674924265279915,-0.01,-0.0109935309893427));
#32629=CARTESIAN_POINT('Origin',(-0.00717019874012884,-0.01000000000001,
-0.010723723701561));
#32630=CARTESIAN_POINT('',(-0.00674924265279915,-0.0155,-0.0109935309893427));
#32631=CARTESIAN_POINT('',(-0.00674924265280681,-0.01000000000001,-0.0109935309893545));
#32632=CARTESIAN_POINT('Origin',(-0.00717019874012884,-0.01550000000001,
-0.010723723701561));
#32633=CARTESIAN_POINT('Origin',(-0.00560796497748951,-0.01,-0.0116172599528138));
#32634=CARTESIAN_POINT('',(-0.00605394934416488,-0.01,-0.011391211407848));
#32635=CARTESIAN_POINT('',(-0.00605394934416488,-0.0155,-0.011391211407848));
#32636=CARTESIAN_POINT('',(-0.00605394934417253,-0.01000000000001,-0.0113912114078599));
#32637=CARTESIAN_POINT('',(-0.00515355568896825,-0.01,-0.011825855730589));
#32638=CARTESIAN_POINT('Origin',(-0.00560796497749716,-0.01000000000001,
-0.0116172599528257));
#32639=CARTESIAN_POINT('',(-0.00515355568896825,-0.0155,-0.011825855730589));
#32640=CARTESIAN_POINT('',(-0.0051535556889759,-0.01000000000001,-0.0118258557306009));
#32641=CARTESIAN_POINT('Origin',(-0.00560796497749716,-0.01550000000001,
-0.0116172599528257));
#32642=CARTESIAN_POINT('Origin',(-0.00393657855553661,-0.01,-0.0122846794535344));
#32643=CARTESIAN_POINT('',(-0.00440968250998357,-0.01,-0.0121228998247591));
#32644=CARTESIAN_POINT('',(-0.00440968250998357,-0.0155,-0.0121228998247591));
#32645=CARTESIAN_POINT('',(-0.00440968250999122,-0.01000000000001,-0.012122899824771));
#32646=CARTESIAN_POINT('',(-0.0034575606257343,-0.01,-0.0124280036417509));
#32647=CARTESIAN_POINT('Origin',(-0.00393657855554426,-0.01000000000001,
-0.0122846794535463));
#32648=CARTESIAN_POINT('',(-0.00345756062573429,-0.0155,-0.0124280036417509));
#32649=CARTESIAN_POINT('',(-0.00345756062574195,-0.01000000000001,-0.0124280036417628));
#32650=CARTESIAN_POINT('Origin',(-0.00393657855554426,-0.01550000000001,
-0.0122846794535463));
#32651=CARTESIAN_POINT('Origin',(-0.00218857110979193,-0.01,-0.0127129916423077));
#32652=CARTESIAN_POINT('',(-0.00267958622168495,-0.01,-0.0126186297861756));
#32653=CARTESIAN_POINT('',(-0.00267958622168495,-0.0155,-0.0126186297861756));
#32654=CARTESIAN_POINT('',(-0.0026795862216926,-0.01000000000001,-0.0126186297861875));
#32655=CARTESIAN_POINT('',(-0.00169426807783735,-0.01,-0.0127882545986707));
#32656=CARTESIAN_POINT('Origin',(-0.00218857110979959,-0.01000000000001,
-0.0127129916423196));
#32657=CARTESIAN_POINT('',(-0.00169426807783735,-0.0155,-0.0127882545986707));
#32658=CARTESIAN_POINT('',(-0.00169426807784501,-0.01000000000001,-0.0127882545986826));
#32659=CARTESIAN_POINT('Origin',(-0.00218857110979959,-0.01550000000001,
-0.0127129916423196));
#32660=CARTESIAN_POINT('Origin',(-0.000397965616857901,-0.01,-0.0128938599095771));
#32661=CARTESIAN_POINT('',(-0.000897334835565383,-0.01,-0.0128687524722826));
#32662=CARTESIAN_POINT('',(-0.000897334835565383,-0.0155,-0.0128687524722826));
#32663=CARTESIAN_POINT('',(-0.000897334835573037,-0.01000000000001,-0.0128687524722945));
#32664=CARTESIAN_POINT('',(0.000102001470993323,-0.01,-0.0128995967262514));
#32665=CARTESIAN_POINT('Origin',(-0.000397965616865556,-0.01000000000001,
-0.012893859909589));
#32666=CARTESIAN_POINT('',(0.000102001470993324,-0.0155,-0.0128995967262514));
#32667=CARTESIAN_POINT('',(0.000102001470985668,-0.01000000000001,-0.0128995967262633));
#32668=CARTESIAN_POINT('Origin',(-0.000397965616865556,-0.01550000000001,
-0.012893859909589));
#32669=CARTESIAN_POINT('Origin',(0.00140038582412907,-0.01,-0.0128237638602548));
#32670=CARTESIAN_POINT('',(0.000902382152425213,-0.01,-0.0128683995295057));
#32671=CARTESIAN_POINT('',(0.000902382152425214,-0.0155,-0.0128683995295057));
#32672=CARTESIAN_POINT('',(0.000902382152417559,-0.01000000000001,-0.0128683995295176));
#32673=CARTESIAN_POINT('',(0.00189628567721606,-0.01,-0.0127598628766294));
#32674=CARTESIAN_POINT('Origin',(0.00140038582412142,-0.01000000000001,
-0.0128237638602667));
#32675=CARTESIAN_POINT('',(0.00189628567721606,-0.0155,-0.0127598628766294));
#32676=CARTESIAN_POINT('',(0.0018962856772084,-0.01000000000001,-0.0127598628766413));
#32677=CARTESIAN_POINT('Origin',(0.00140038582412142,-0.01550000000001,
-0.0128237638602667));
#32678=CARTESIAN_POINT('Origin',(0.00317148034796465,-0.01,-0.0125040678342079));
#32679=CARTESIAN_POINT('',(0.00268453529826336,-0.01,-0.0126175778274746));
#32680=CARTESIAN_POINT('',(0.00268453529826336,-0.0155,-0.0126175778274746));
#32681=CARTESIAN_POINT('',(0.0026845352982557,-0.01000000000001,-0.0126175778274865));
#32682=CARTESIAN_POINT('',(0.0036536608397248,-0.01,-0.0123717728102428));
#32683=CARTESIAN_POINT('Origin',(0.00317148034797655,-0.01000000000001,
-0.0125040678342156));
#32684=CARTESIAN_POINT('',(0.0036536608397248,-0.0155,-0.0123717728102428));
#32685=CARTESIAN_POINT('',(0.00365366083973669,-0.01000000000001,-0.0123717728102504));
#32686=CARTESIAN_POINT('Origin',(0.00317148034797655,-0.01550000000001,
-0.0125040678342156));
#32687=CARTESIAN_POINT('Origin',(0.00488084561433254,-0.01,-0.0119409943509345));
#32688=CARTESIAN_POINT('',(0.00441443701813444,-0.01,-0.0121211693253137));
#32689=CARTESIAN_POINT('',(0.00441443701813444,-0.0155,-0.0121211693253137));
#32690=CARTESIAN_POINT('',(0.00441443701814632,-0.01000000000001,-0.0121211693253213));
#32691=CARTESIAN_POINT('',(0.00533992164996587,-0.01,-0.0117428802587877));
#32692=CARTESIAN_POINT('Origin',(0.00488084561434443,-0.01000000000001,
-0.0119409943509422));
#32693=CARTESIAN_POINT('',(0.00533992164996587,-0.0155,-0.0117428802587877));
#32694=CARTESIAN_POINT('',(0.00533992164997777,-0.01000000000001,-0.0117428802587953));
#32695=CARTESIAN_POINT('Origin',(0.00488084561434443,-0.01550000000001,
-0.0119409943509422));
#32696=CARTESIAN_POINT('Origin',(0.00649521077269703,-0.01,-0.0111455029953));
#32697=CARTESIAN_POINT('',(0.00605841674279519,-0.01,-0.0113888360498612));
#32698=CARTESIAN_POINT('',(0.00605841674279519,-0.0155,-0.0113888360498612));
#32699=CARTESIAN_POINT('',(0.00605841674280708,-0.01000000000001,-0.0113888360498688));
#32700=CARTESIAN_POINT('',(0.00692224695936122,-0.01,-0.0108854259004236));
#32701=CARTESIAN_POINT('Origin',(0.00649521077270892,-0.01000000000001,
-0.0111455029953076));
#32702=CARTESIAN_POINT('',(0.00692224695936122,-0.0155,-0.0108854259004236));
#32703=CARTESIAN_POINT('',(0.00692224695937311,-0.01000000000001,-0.0108854259004312));
#32704=CARTESIAN_POINT('Origin',(0.00649521077270892,-0.01550000000001,
-0.0111455029953076));
#32705=CARTESIAN_POINT('Origin',(0.00798315404156373,-0.01,-0.0101330771016836));
#32706=CARTESIAN_POINT('',(0.00758447627690437,-0.01,-0.0104348320353073));
#32707=CARTESIAN_POINT('',(0.00758447627690437,-0.0155,-0.0104348320353073));
#32708=CARTESIAN_POINT('',(0.00758447627691625,-0.01000000000001,-0.0104348320353149));
#32709=CARTESIAN_POINT('',(0.00836983860563182,-0.01,-0.0098160991088963));
#32710=CARTESIAN_POINT('Origin',(0.00798315404157562,-0.01000000000001,
-0.0101330771016913));
#32711=CARTESIAN_POINT('',(0.00836983860563182,-0.0155,-0.0098160991088963));
#32712=CARTESIAN_POINT('',(0.00836983860564371,-0.01000000000001,-0.00981609910890396));
#32713=CARTESIAN_POINT('Origin',(0.00798315404157562,-0.01550000000001,
-0.0101330771016913));
#32714=CARTESIAN_POINT('Origin',(0.00931571429771449,-0.01,-0.00892342238848729));
#32715=CARTESIAN_POINT('',(0.00896291260749749,-0.01,-0.00927772588463158));
#32716=CARTESIAN_POINT('',(0.00896291260749749,-0.0155,-0.00927772588463158));
#32717=CARTESIAN_POINT('',(0.00896291260750937,-0.01000000000001,-0.00927772588463924));
#32718=CARTESIAN_POINT('',(0.00965452086399409,-0.01,-0.00855571311386156));
#32719=CARTESIAN_POINT('Origin',(0.00931571429772638,-0.01000000000001,
-0.00892342238849495));
#32720=CARTESIAN_POINT('',(0.00965452086399409,-0.0155,-0.00855571311386156));
#32721=CARTESIAN_POINT('',(0.00965452086400598,-0.01000000000001,-0.00855571311386922));
#32722=CARTESIAN_POINT('Origin',(0.00931571429772638,-0.01550000000001,
-0.00892342238849495));
#32723=CARTESIAN_POINT('Origin',(0.0104669547715282,-0.01,-0.00754008340874168));
#32724=CARTESIAN_POINT('',(0.0101668960393476,-0.01,-0.00794003935286826));
#32725=CARTESIAN_POINT('',(0.0101668960393476,-0.0155,-0.00794003935286826));
#32726=CARTESIAN_POINT('',(0.0101668960393595,-0.01000000000001,-0.00794003935287591));
#32727=CARTESIAN_POINT('',(0.0107512888555934,-0.01,-0.00712879989504486));
#32728=CARTESIAN_POINT('Origin',(0.0104669547715401,-0.01000000000001,-0.00754008340874933));
#32729=CARTESIAN_POINT('',(0.0107512888555934,-0.0155,-0.00712879989504486));
#32730=CARTESIAN_POINT('',(0.0107512888556053,-0.01000000000001,-0.00712879989505252));
#32731=CARTESIAN_POINT('Origin',(0.0104669547715401,-0.01550000000001,-0.00754008340874933));
#32732=CARTESIAN_POINT('Origin',(0.0114144678766987,-0.01,-0.00600998528216265));
#32733=CARTESIAN_POINT('',(0.0111729924044647,-0.01,-0.00644780898676229));
#32734=CARTESIAN_POINT('',(0.0111729924044647,-0.0155,-0.00644780898676229));
#32735=CARTESIAN_POINT('',(0.0111729924044766,-0.01000000000001,-0.00644780898676994));
#32736=CARTESIAN_POINT('',(0.0116387952390284,-0.01,-0.00556313269516086));
#32737=CARTESIAN_POINT('Origin',(0.0114144678767106,-0.01000000000001,-0.0060099852821703));
#32738=CARTESIAN_POINT('',(0.0116387952390284,-0.0155,-0.00556313269516086));
#32739=CARTESIAN_POINT('',(0.0116387952390403,-0.01000000000001,-0.00556313269516851));
#32740=CARTESIAN_POINT('Origin',(0.0114144678767106,-0.01550000000001,-0.0060099852821703));
#32741=CARTESIAN_POINT('Origin',(0.0121398113484141,-0.01,-0.00436290962832323));
#32742=CARTESIAN_POINT('',(0.0119616191815194,-0.01,-0.004830079353003));
#32743=CARTESIAN_POINT('',(0.0119616191815194,-0.0155,-0.004830079353003));
#32744=CARTESIAN_POINT('',(0.0119616191815313,-0.01000000000001,-0.00483007935301066));
#32745=CARTESIAN_POINT('',(0.0122997657120691,-0.01,-0.00388918544533519));
#32746=CARTESIAN_POINT('Origin',(0.012139811348426,-0.01000000000001,-0.00436290962833088));
#32747=CARTESIAN_POINT('',(0.0122997657120691,-0.0155,-0.00388918544533519));
#32748=CARTESIAN_POINT('',(0.012299765712081,-0.01000000000001,-0.00388918544534284));
#32749=CARTESIAN_POINT('Origin',(0.012139811348426,-0.01550000000001,-0.00436290962833088));
#32750=CARTESIAN_POINT('Origin',(0.0126288672010633,-0.01,-0.00263091490130466));
#32751=CARTESIAN_POINT('',(0.012517426647346,-0.01,-0.00311833771877137));
#32752=CARTESIAN_POINT('',(0.012517426647346,-0.0155,-0.00311833771877137));
#32753=CARTESIAN_POINT('',(0.0125174266473579,-0.01000000000001,-0.00311833771877902));
#32754=CARTESIAN_POINT('',(0.0127213352363006,-0.01,-0.00213953962469893));
#32755=CARTESIAN_POINT('Origin',(0.0126288672010752,-0.01000000000001,-0.00263091490131231));
#32756=CARTESIAN_POINT('',(0.0127213352363006,-0.0155,-0.00213953962469893));
#32757=CARTESIAN_POINT('',(0.0127213352363125,-0.01000000000001,-0.00213953962470658));
#32758=CARTESIAN_POINT('Origin',(0.0126288672010752,-0.01550000000001,-0.00263091490131231));
#32759=CARTESIAN_POINT('Origin',(0.0128721165187673,-0.01,-0.000847712408353549));
#32760=CARTESIAN_POINT('',(0.0128295966418437,-0.01,-0.00134590118790042));
#32761=CARTESIAN_POINT('',(0.0128295966418437,-0.0155,-0.00134590118790042));
#32762=CARTESIAN_POINT('',(0.0128295966418555,-0.01000000000001,-0.00134590118790808));
#32763=CARTESIAN_POINT('',(0.0128952984404617,-0.01,-0.000348250098958184));
#32764=CARTESIAN_POINT('Origin',(0.0128721165187792,-0.01000000000001,-0.000847712408361203));
#32765=CARTESIAN_POINT('',(0.0128952984404617,-0.0155,-0.000348250098958184));
#32766=CARTESIAN_POINT('',(0.0128952984404736,-0.01000000000001,-0.000348250098965837));
#32767=CARTESIAN_POINT('Origin',(0.0128721165187792,-0.01550000000001,-0.000847712408361203));
#32768=CARTESIAN_POINT('Origin',(0.0128648247302491,-0.01,0.000951989842367618));
#32769=CARTESIAN_POINT('',(0.0128920531311578,-0.01,0.000452731778653103));
#32770=CARTESIAN_POINT('',(0.0128920531311578,-0.0155,0.000452731778653103));
#32771=CARTESIAN_POINT('',(0.0128920531311697,-0.01000000000001,0.000452731778645449));
#32772=CARTESIAN_POINT('',(0.0128182693286638,-0.01,0.00144981771883018));
#32773=CARTESIAN_POINT('Origin',(0.012864824730261,-0.01000000000001,0.000951989842359964));
#32774=CARTESIAN_POINT('',(0.0128182693286638,-0.0155,0.00144981771883019));
#32775=CARTESIAN_POINT('',(0.0128182693286757,-0.01000000000001,0.00144981771882252));
#32776=CARTESIAN_POINT('Origin',(0.012864824730261,-0.01550000000001,0.000951989842359964));
#32777=CARTESIAN_POINT('Origin',(-4.47228396786959E-17,-0.01,1.11925812962326E-32));
#32778=CARTESIAN_POINT('',(0.0124917471849488,-0.01,0.00321966648386474));
#32779=CARTESIAN_POINT('Origin',(-4.47228396786953E-17,-0.01000000000001,
1.11925812962343E-32));
#32780=CARTESIAN_POINT('',(0.0127035804707671,-0.01,0.00224255283610991));
#32781=CARTESIAN_POINT('Origin',(0.0126071337618875,-0.01000000000001,0.00273316269368159));
#32782=CARTESIAN_POINT('Origin',(-4.47228396786953E-17,-0.01000000000001,
1.11925812962343E-32));
#32783=CARTESIAN_POINT('Origin',(-4.47228396786953E-17,-0.01000000000001,
1.11925812962343E-32));
#32784=CARTESIAN_POINT('Origin',(-4.47228396786953E-17,-0.01000000000001,
1.11925812962343E-32));
#32785=CARTESIAN_POINT('Origin',(-4.47228396786953E-17,-0.01000000000001,
1.11925812962343E-32));
#32786=CARTESIAN_POINT('Origin',(-4.47228396786953E-17,-0.01000000000001,
1.11925812962343E-32));
#32787=CARTESIAN_POINT('Origin',(-4.47228396786953E-17,-0.01000000000001,
1.11925812962343E-32));
#32788=CARTESIAN_POINT('Origin',(-4.47228396786953E-17,-0.01000000000001,
1.11925812962343E-32));
#32789=CARTESIAN_POINT('Origin',(-4.47228396786953E-17,-0.01000000000001,
1.11925812962343E-32));
#32790=CARTESIAN_POINT('Origin',(-4.47228396786953E-17,-0.01000000000001,
1.11925812962343E-32));
#32791=CARTESIAN_POINT('Origin',(-4.47228396786953E-17,-0.01000000000001,
1.11925812962343E-32));
#32792=CARTESIAN_POINT('Origin',(-4.47228396786953E-17,-0.01000000000001,
1.11925812962343E-32));
#32793=CARTESIAN_POINT('Origin',(-4.47228396786953E-17,-0.01000000000001,
1.11925812962343E-32));
#32794=CARTESIAN_POINT('Origin',(-4.47228396786953E-17,-0.01000000000001,
1.11925812962343E-32));
#32795=CARTESIAN_POINT('Origin',(-4.47228396786953E-17,-0.01000000000001,
1.11925812962343E-32));
#32796=CARTESIAN_POINT('Origin',(-4.47228396786953E-17,-0.01000000000001,
1.11925812962343E-32));
#32797=CARTESIAN_POINT('Origin',(-4.47228396786953E-17,-0.01000000000001,
1.11925812962343E-32));
#32798=CARTESIAN_POINT('Origin',(-4.47228396786953E-17,-0.01000000000001,
1.11925812962343E-32));
#32799=CARTESIAN_POINT('Origin',(-4.47228396786953E-17,-0.01000000000001,
1.11925812962343E-32));
#32800=CARTESIAN_POINT('Origin',(-4.47228396786953E-17,-0.01000000000001,
1.11925812962343E-32));
#32801=CARTESIAN_POINT('Origin',(-4.47228396786953E-17,-0.01000000000001,
1.11925812962343E-32));
#32802=CARTESIAN_POINT('Origin',(-4.47228396786953E-17,-0.01000000000001,
1.11925812962343E-32));
#32803=CARTESIAN_POINT('Origin',(-4.47228396786953E-17,-0.01000000000001,
1.11925812962343E-32));
#32804=CARTESIAN_POINT('Origin',(-4.47228396786953E-17,-0.01000000000001,
1.11925812962343E-32));
#32805=CARTESIAN_POINT('Origin',(-4.47228396786953E-17,-0.01000000000001,
1.11925812962343E-32));
#32806=CARTESIAN_POINT('Origin',(-4.47228396786953E-17,-0.01000000000001,
1.11925812962343E-32));
#32807=CARTESIAN_POINT('Origin',(-4.47228396786953E-17,-0.01000000000001,
1.11925812962343E-32));
#32808=CARTESIAN_POINT('Origin',(-4.47228396786953E-17,-0.01000000000001,
1.11925812962343E-32));
#32809=CARTESIAN_POINT('Origin',(-4.47228396786953E-17,-0.01000000000001,
1.11925812962343E-32));
#32810=CARTESIAN_POINT('Origin',(-4.47228396786953E-17,-0.01000000000001,
1.11925812962343E-32));
#32811=CARTESIAN_POINT('Origin',(-4.47228396786953E-17,-0.01000000000001,
1.11925812962343E-32));
#32812=CARTESIAN_POINT('Origin',(-4.47228396786953E-17,-0.01000000000001,
1.11925812962343E-32));
#32813=CARTESIAN_POINT('Origin',(-4.47228396786953E-17,-0.01000000000001,
1.11925812962343E-32));
#32814=CARTESIAN_POINT('Origin',(-4.47228396786953E-17,-0.01000000000001,
1.11925812962343E-32));
#32815=CARTESIAN_POINT('Origin',(-4.47228396786953E-17,-0.01000000000001,
1.11925812962343E-32));
#32816=CARTESIAN_POINT('Origin',(-4.47228396786953E-17,-0.01000000000001,
1.11925812962343E-32));
#32817=CARTESIAN_POINT('Origin',(-4.47228396786953E-17,-0.01000000000001,
1.11925812962343E-32));
#32818=CARTESIAN_POINT('Origin',(-4.47228396786953E-17,-0.01000000000001,
1.11925812962343E-32));
#32819=CARTESIAN_POINT('Origin',(-4.47228396786953E-17,-0.01000000000001,
1.11925812962343E-32));
#32820=CARTESIAN_POINT('Origin',(-4.47228396786953E-17,-0.01000000000001,
1.11925812962343E-32));
#32821=CARTESIAN_POINT('Origin',(-4.47228396786953E-17,-0.01000000000001,
1.11925812962343E-32));
#32822=CARTESIAN_POINT('Origin',(-4.47228396786953E-17,-0.01000000000001,
1.11925812962343E-32));
#32823=CARTESIAN_POINT('Origin',(-4.47228396786953E-17,-0.01000000000001,
1.11925812962343E-32));
#32824=CARTESIAN_POINT('Origin',(-4.47228396786953E-17,-0.01000000000001,
1.11925812962343E-32));
#32825=CARTESIAN_POINT('Origin',(-4.47228396786953E-17,-0.01000000000001,
1.11925812962343E-32));
#32826=CARTESIAN_POINT('',(-0.000529682692573584,-0.01000000000001,0.0024432429771081));
#32827=CARTESIAN_POINT('Origin',(-4.47228396786953E-17,-0.01000000000001,
1.11925812962343E-32));
#32828=CARTESIAN_POINT('Origin',(-4.43566503645872E-17,-0.0155,1.21332054810713E-32));
#32829=CARTESIAN_POINT('',(0.0124917471849488,-0.0155,0.00321966648386474));
#32830=CARTESIAN_POINT('Origin',(-4.43566503645865E-17,-0.01550000000001,
1.21332054810731E-32));
#32831=CARTESIAN_POINT('',(0.0124917471849565,-0.01000000000001,0.00321966648387663));
#32832=CARTESIAN_POINT('Origin',(-4.43566503645872E-17,-0.0155,1.21332054810713E-32));
#32833=CARTESIAN_POINT('',(0.0127035804707671,-0.0155,0.00224255283610991));
#32834=CARTESIAN_POINT('',(0.012703580470779,-0.01000000000001,0.00224255283610226));
#32835=CARTESIAN_POINT('Origin',(-4.43566503645865E-17,-0.01550000000001,
1.21332054810731E-32));
#32836=CARTESIAN_POINT('Origin',(-4.43566503645872E-17,-0.0155,1.21332054810713E-32));
#32837=CARTESIAN_POINT('Origin',(-4.43566503645865E-17,-0.01550000000001,
1.21332054810731E-32));
#32838=CARTESIAN_POINT('Origin',(-4.43566503645872E-17,-0.0155,1.21332054810713E-32));
#32839=CARTESIAN_POINT('Origin',(-4.43566503645865E-17,-0.01550000000001,
1.21332054810731E-32));
#32840=CARTESIAN_POINT('Origin',(-4.43566503645872E-17,-0.0155,1.21332054810713E-32));
#32841=CARTESIAN_POINT('Origin',(-4.43566503645865E-17,-0.01550000000001,
1.21332054810731E-32));
#32842=CARTESIAN_POINT('Origin',(-4.43566503645872E-17,-0.0155,1.21332054810713E-32));
#32843=CARTESIAN_POINT('Origin',(-4.43566503645865E-17,-0.01550000000001,
1.21332054810731E-32));
#32844=CARTESIAN_POINT('Origin',(-4.43566503645872E-17,-0.0155,1.21332054810713E-32));
#32845=CARTESIAN_POINT('Origin',(-4.43566503645865E-17,-0.01550000000001,
1.21332054810731E-32));
#32846=CARTESIAN_POINT('Origin',(-4.43566503645872E-17,-0.0155,1.21332054810713E-32));
#32847=CARTESIAN_POINT('Origin',(-4.43566503645865E-17,-0.01550000000001,
1.21332054810731E-32));
#32848=CARTESIAN_POINT('Origin',(-4.43566503645872E-17,-0.0155,1.21332054810713E-32));
#32849=CARTESIAN_POINT('Origin',(-4.43566503645865E-17,-0.01550000000001,
1.21332054810731E-32));
#32850=CARTESIAN_POINT('Origin',(-4.43566503645872E-17,-0.0155,1.21332054810713E-32));
#32851=CARTESIAN_POINT('Origin',(-4.43566503645865E-17,-0.01550000000001,
1.21332054810731E-32));
#32852=CARTESIAN_POINT('Origin',(-4.43566503645872E-17,-0.0155,1.21332054810713E-32));
#32853=CARTESIAN_POINT('Origin',(-4.43566503645865E-17,-0.01550000000001,
1.21332054810731E-32));
#32854=CARTESIAN_POINT('Origin',(-4.43566503645872E-17,-0.0155,1.21332054810713E-32));
#32855=CARTESIAN_POINT('Origin',(-4.43566503645865E-17,-0.01550000000001,
1.21332054810731E-32));
#32856=CARTESIAN_POINT('Origin',(-4.43566503645872E-17,-0.0155,1.21332054810713E-32));
#32857=CARTESIAN_POINT('Origin',(-4.43566503645865E-17,-0.01550000000001,
1.21332054810731E-32));
#32858=CARTESIAN_POINT('Origin',(-4.43566503645872E-17,-0.0155,1.21332054810713E-32));
#32859=CARTESIAN_POINT('Origin',(-4.43566503645865E-17,-0.01550000000001,
1.21332054810731E-32));
#32860=CARTESIAN_POINT('Origin',(-4.43566503645872E-17,-0.0155,1.21332054810713E-32));
#32861=CARTESIAN_POINT('Origin',(-4.43566503645865E-17,-0.01550000000001,
1.21332054810731E-32));
#32862=CARTESIAN_POINT('Origin',(-4.43566503645872E-17,-0.0155,1.21332054810713E-32));
#32863=CARTESIAN_POINT('Origin',(-4.43566503645865E-17,-0.01550000000001,
1.21332054810731E-32));
#32864=CARTESIAN_POINT('Origin',(-4.43566503645872E-17,-0.0155,1.21332054810713E-32));
#32865=CARTESIAN_POINT('Origin',(-4.43566503645865E-17,-0.01550000000001,
1.21332054810731E-32));
#32866=CARTESIAN_POINT('Origin',(-4.43566503645872E-17,-0.0155,1.21332054810713E-32));
#32867=CARTESIAN_POINT('Origin',(-4.43566503645865E-17,-0.01550000000001,
1.21332054810731E-32));
#32868=CARTESIAN_POINT('Origin',(-4.43566503645872E-17,-0.0155,1.21332054810713E-32));
#32869=CARTESIAN_POINT('Origin',(-4.43566503645865E-17,-0.01550000000001,
1.21332054810731E-32));
#32870=CARTESIAN_POINT('Origin',(-4.43566503645872E-17,-0.0155,1.21332054810713E-32));
#32871=CARTESIAN_POINT('Origin',(-4.43566503645865E-17,-0.01550000000001,
1.21332054810731E-32));
#32872=CARTESIAN_POINT('Origin',(-4.43566503645872E-17,-0.0155,1.21332054810713E-32));
#32873=CARTESIAN_POINT('Origin',(-4.43566503645865E-17,-0.01550000000001,
1.21332054810731E-32));
#32874=CARTESIAN_POINT('Origin',(-4.43566503645872E-17,-0.0155,1.21332054810713E-32));
#32875=CARTESIAN_POINT('Origin',(-4.43566503645865E-17,-0.01550000000001,
1.21332054810731E-32));
#32876=CARTESIAN_POINT('Origin',(-4.43566503645872E-17,-0.0155,1.21332054810713E-32));
#32877=CARTESIAN_POINT('Origin',(-4.43566503645865E-17,-0.01550000000001,
1.21332054810731E-32));
#32878=CARTESIAN_POINT('Origin',(-4.43566503645872E-17,-0.0155,1.21332054810713E-32));
#32879=CARTESIAN_POINT('Origin',(-4.43566503645865E-17,-0.01550000000001,
1.21332054810731E-32));
#32880=CARTESIAN_POINT('Origin',(-4.43566503645872E-17,-0.0155,1.21332054810713E-32));
#32881=CARTESIAN_POINT('Origin',(-4.43566503645865E-17,-0.01550000000001,
1.21332054810731E-32));
#32882=CARTESIAN_POINT('Origin',(-4.43566503645872E-17,-0.0155,1.21332054810713E-32));
#32883=CARTESIAN_POINT('Origin',(-4.43566503645865E-17,-0.01550000000001,
1.21332054810731E-32));
#32884=CARTESIAN_POINT('Origin',(-4.43566503645872E-17,-0.0155,1.21332054810713E-32));
#32885=CARTESIAN_POINT('Origin',(-4.43566503645865E-17,-0.01550000000001,
1.21332054810731E-32));
#32886=CARTESIAN_POINT('Origin',(-4.43566503645872E-17,-0.0155,1.21332054810713E-32));
#32887=CARTESIAN_POINT('Origin',(-4.43566503645865E-17,-0.01550000000001,
1.21332054810731E-32));
#32888=CARTESIAN_POINT('Origin',(-4.43566503645872E-17,-0.0155,1.21332054810713E-32));
#32889=CARTESIAN_POINT('Origin',(-4.43566503645865E-17,-0.01550000000001,
1.21332054810731E-32));
#32890=CARTESIAN_POINT('Origin',(-4.43566503645872E-17,-0.0155,1.21332054810713E-32));
#32891=CARTESIAN_POINT('Origin',(-4.43566503645865E-17,-0.01550000000001,
1.21332054810731E-32));
#32892=CARTESIAN_POINT('Origin',(-4.43566503645872E-17,-0.0155,1.21332054810713E-32));
#32893=CARTESIAN_POINT('Origin',(-4.43566503645865E-17,-0.01550000000001,
1.21332054810731E-32));
#32894=CARTESIAN_POINT('Origin',(-4.43566503645872E-17,-0.0155,1.21332054810713E-32));
#32895=CARTESIAN_POINT('Origin',(-4.43566503645865E-17,-0.01550000000001,
1.21332054810731E-32));
#32896=CARTESIAN_POINT('Origin',(-4.43566503645872E-17,-0.0155,1.21332054810713E-32));
#32897=CARTESIAN_POINT('Origin',(-4.43566503645865E-17,-0.01550000000001,
1.21332054810731E-32));
#32898=CARTESIAN_POINT('Origin',(-4.43566503645872E-17,-0.0155,1.21332054810713E-32));
#32899=CARTESIAN_POINT('Origin',(-4.43566503645865E-17,-0.01550000000001,
1.21332054810731E-32));
#32900=CARTESIAN_POINT('Origin',(-4.43566503645872E-17,-0.0155,1.21332054810713E-32));
#32901=CARTESIAN_POINT('Origin',(-4.43566503645865E-17,-0.01550000000001,
1.21332054810731E-32));
#32902=CARTESIAN_POINT('Origin',(-4.43566503645872E-17,-0.0155,1.21332054810713E-32));
#32903=CARTESIAN_POINT('Origin',(-4.43566503645865E-17,-0.01550000000001,
1.21332054810731E-32));
#32904=CARTESIAN_POINT('Origin',(-4.43566503645872E-17,-0.0155,1.21332054810713E-32));
#32905=CARTESIAN_POINT('Origin',(-4.43566503645865E-17,-0.01550000000001,
1.21332054810731E-32));
#32906=CARTESIAN_POINT('Origin',(-4.43566503645872E-17,-0.0155,1.21332054810713E-32));
#32907=CARTESIAN_POINT('Origin',(-4.43566503645865E-17,-0.01550000000001,
1.21332054810731E-32));
#32908=CARTESIAN_POINT('Origin',(-4.43566503645872E-17,-0.0155,1.21332054810713E-32));
#32909=CARTESIAN_POINT('Origin',(-4.43566503645865E-17,-0.01550000000001,
1.21332054810731E-32));
#32910=CARTESIAN_POINT('Origin',(-4.43566503645872E-17,-0.0155,1.21332054810713E-32));
#32911=CARTESIAN_POINT('Origin',(-4.43566503645865E-17,-0.01550000000001,
1.21332054810731E-32));
#32912=CARTESIAN_POINT('Origin',(-4.43566503645872E-17,-0.0155,1.21332054810713E-32));
#32913=CARTESIAN_POINT('Origin',(-4.43566503645865E-17,-0.01550000000001,
1.21332054810731E-32));
#32914=CARTESIAN_POINT('Origin',(-4.43566503645872E-17,-0.0155,1.21332054810713E-32));
#32915=CARTESIAN_POINT('Origin',(-4.43566503645865E-17,-0.01550000000001,
1.21332054810731E-32));
#32916=CARTESIAN_POINT('Origin',(-4.43566503645872E-17,-0.0155,1.21332054810713E-32));
#32917=CARTESIAN_POINT('Origin',(-4.43566503645865E-17,-0.01550000000001,
1.21332054810731E-32));
#32918=CARTESIAN_POINT('Origin',(-4.43566503645872E-17,-0.0155,1.21332054810713E-32));
#32919=CARTESIAN_POINT('Origin',(-4.43566503645865E-17,-0.01550000000001,
1.21332054810731E-32));
#32920=CARTESIAN_POINT('Origin',(0.0126071337618777,-0.01,0.00273316269367947));
#32921=CARTESIAN_POINT('Origin',(0.0126071337618875,-0.01550000000001,0.00273316269368159));
#32922=CARTESIAN_POINT('Origin',(-4.43566503645872E-17,-0.0155,1.21332054810713E-32));
#32923=CARTESIAN_POINT('Origin',(-4.43566503645865E-17,-0.01550000000001,
1.21332054810731E-32));
#32924=CARTESIAN_POINT('',(-0.000529682692573584,-0.01550000000001,0.0024432429771081));
#32925=CARTESIAN_POINT('Origin',(-4.43566503645865E-17,-0.01550000000001,
1.21332054810731E-32));
#32926=CARTESIAN_POINT('Origin',(-4.43566503645872E-17,-0.0155,1.21332054810713E-32));
#32927=CARTESIAN_POINT('Origin',(-4.43566503645872E-17,-0.0155,1.21332054810713E-32));
#32928=CARTESIAN_POINT('',(-0.000529682692573584,-0.0155,0.0024432429771081));
#34828=UNCERTAINTY_MEASURE_WITH_UNIT(LENGTH_MEASURE(1.E-5),#34877,
'DISTANCE_ACCURACY_VALUE',
'Maximum model space distance between geometric entities at asserted c
onnectivities');
#34841=UNCERTAINTY_MEASURE_WITH_UNIT(LENGTH_MEASURE(1.E-5),#34877,
'DISTANCE_ACCURACY_VALUE',
'Maximum model space distance between geometric entities at asserted c
onnectivities');
#34863=(
GEOMETRIC_REPRESENTATION_CONTEXT(3)
GLOBAL_UNCERTAINTY_ASSIGNED_CONTEXT((#34828))
GLOBAL_UNIT_ASSIGNED_CONTEXT((#34877,#34878,#34879))
REPRESENTATION_CONTEXT('','3D')
);
#34876=(
GEOMETRIC_REPRESENTATION_CONTEXT(3)
GLOBAL_UNCERTAINTY_ASSIGNED_CONTEXT((#34841))
GLOBAL_UNIT_ASSIGNED_CONTEXT((#34877,#34878,#34879))
REPRESENTATION_CONTEXT('','3D')
);
#34877=(
LENGTH_UNIT()
NAMED_UNIT(*)
SI_UNIT($,.METRE.)
);
#34878=(
NAMED_UNIT(*)
PLANE_ANGLE_UNIT()
SI_UNIT($,.RADIAN.)
);
#34879=(
NAMED_UNIT(*)
SI_UNIT($,.STERADIAN.)
SOLID_ANGLE_UNIT()
);
#34901=SHAPE_DEFINITION_REPRESENTATION(#34935,#35005);
#34935=PRODUCT_DEFINITION_SHAPE('',$,#35040);
#35005=SHAPE_REPRESENTATION('',(#21374),#34863);
#35018=PRODUCT_DEFINITION_CONTEXT('part definition',#35122,'design');
#35040=PRODUCT_DEFINITION('Motor Shaft 3','Motor Shaft 3',#35074,#35018);
#35074=PRODUCT_DEFINITION_FORMATION('',$,#35145);
#35122=APPLICATION_CONTEXT('Managed model based 3d engineering');
#35123=PRODUCT_CONTEXT('part definition',#35122,'mechanical');
#35145=PRODUCT('Motor Shaft 3','Motor Shaft 3',
'LEGAL AND USAGE DISCLAIMER: this Data/Model is provided \X2\201C\X0\A
S IS\X2\201D\X0\ for informational and representational only. It is a 
geometric approximation and is NOT engineered, certified, or guarantee
d for dimensional accuracy, exact tolerances, or production-level prec
ision. Vendor disclaims all implied warranties including fitness for a
 particular purpose. DO NOT USE FOR DIRECT PHYSICAL MANUFACTURING, AUT
OMATED PRODUCTION, OR SAFETY-CRITICAL SYSTEMS without independent engi
neering verification and resolution of any design discrepancies.',(#35123));
#35161=PRESENTATION_STYLE_ASSIGNMENT((#35170));
#35170=SURFACE_STYLE_USAGE(.BOTH.,#35179);
#35179=SURFACE_SIDE_STYLE('',(#35188));
#35188=SURFACE_STYLE_FILL_AREA(#35197);
#35197=FILL_AREA_STYLE('Aluminum - Anodized Glossy (Blue)',(#35206));
#35206=FILL_AREA_STYLE_COLOUR('Aluminum - Anodized Glossy (Blue)',#35215);
#35215=COLOUR_RGB('Aluminum - Anodized Glossy (Blue)',0.349019607843137,
0.584313725490196,0.854901960784314);
ENDSEC;
END-ISO-10303-21;
